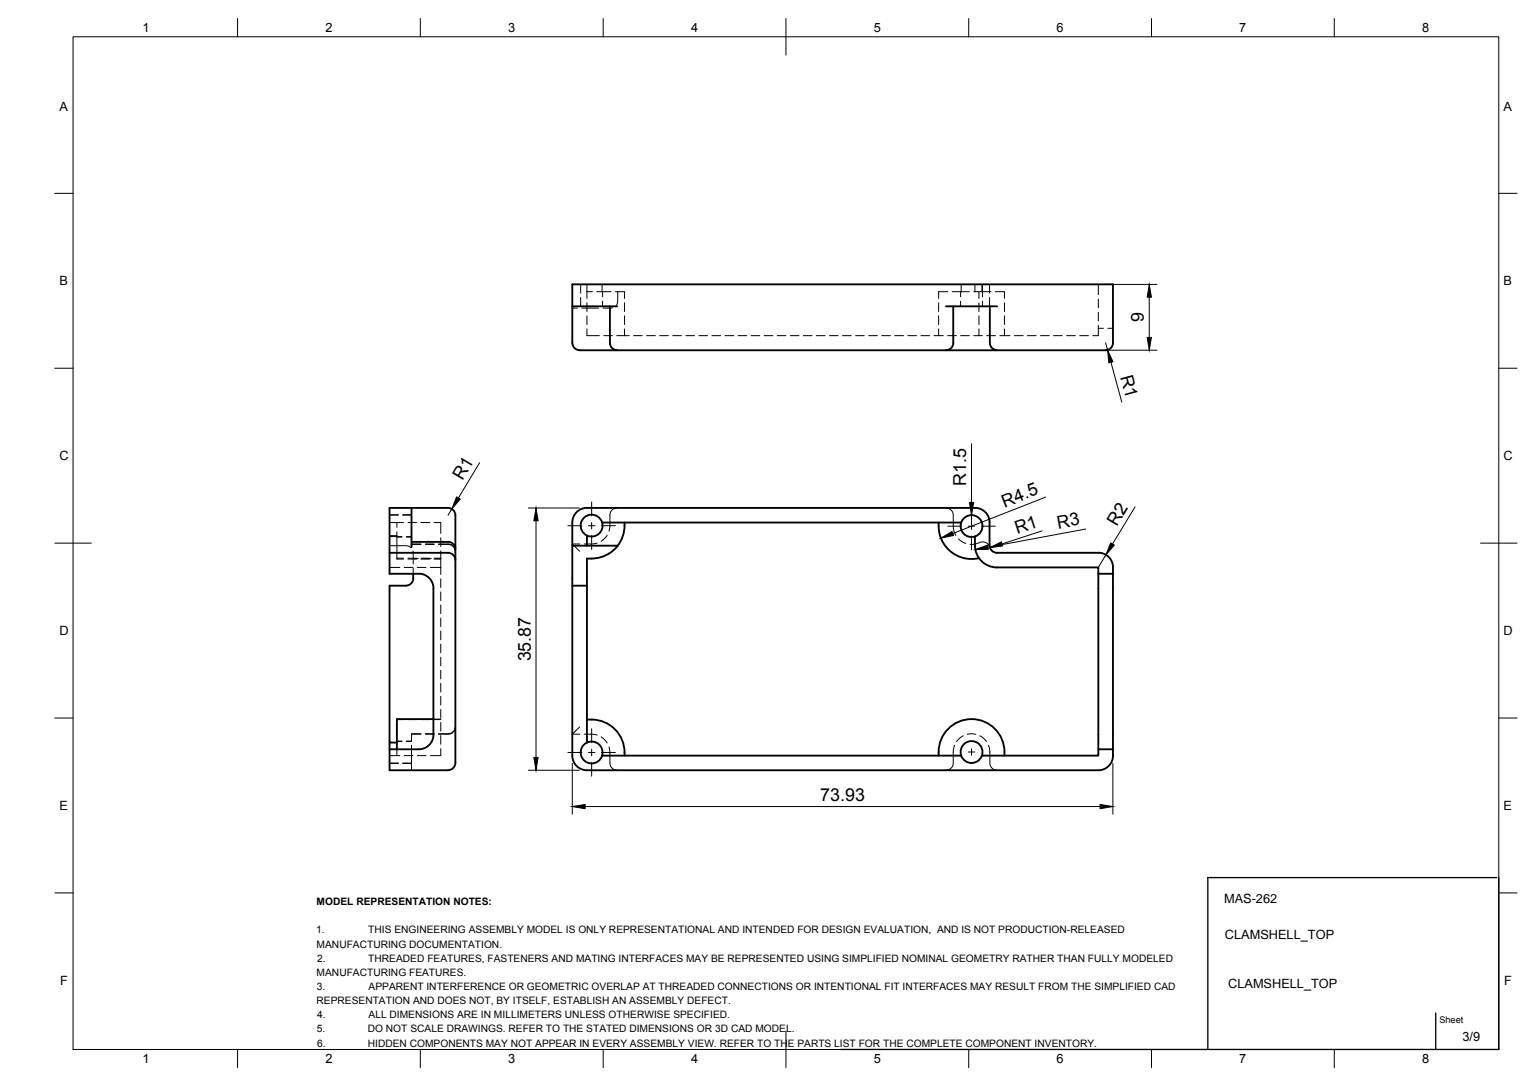
ISO-10303-21;
HEADER;
/* Generated by software containing ST-Developer
 * from STEP Tools, Inc. (www.steptools.com) 
 */

FILE_DESCRIPTION(
/* description */ (''),
/* implementation_level */ '2;1');

FILE_NAME(
/* name */ 'CLAMSHELL_TOP.step',
/* time_stamp */ '2026-10-07T02:13:48+06:00',
/* author */ (''),
/* organization */ (''),
/* preprocessor_version */ 'ST-DEVELOPER v20.2',
/* originating_system */ 'Autodesk Translation Framework v15.15.0.0',
/* authorisation */ '');

FILE_SCHEMA (('AUTOMOTIVE_DESIGN { 1 0 10303 214 3 1 1 }'));
ENDSEC;

DATA;
#10=MECHANICAL_DESIGN_GEOMETRIC_PRESENTATION_REPRESENTATION('',(#114),#17042);
#90=SHAPE_REPRESENTATION_RELATIONSHIP('SRR','None',#17086,#102);
#102=ADVANCED_BREP_SHAPE_REPRESENTATION('',(#126),#17030);
#114=STYLED_ITEM('',(#17154),#126);
#126=MANIFOLD_SOLID_BREP('Body1',#8115);
#138=FACE_BOUND('',#1043,.T.);
#139=FACE_BOUND('',#1045,.T.);
#140=FACE_BOUND('',#1050,.T.);
#141=FACE_BOUND('',#1052,.T.);
#178=(
BOUNDED_SURFACE()
B_SPLINE_SURFACE(2,2,((#12260,#12261,#12262),(#12263,#12264,#12265),(#12266,
#12267,#12268)),.UNSPECIFIED.,.F.,.F.,.F.)
B_SPLINE_SURFACE_WITH_KNOTS((3,3),(3,3),(-1.5707963267949,0.),(0.,1.5707963267949),
 .UNSPECIFIED.)
GEOMETRIC_REPRESENTATION_ITEM()
RATIONAL_B_SPLINE_SURFACE(((1.,0.707106781186548,1.),(0.707106781186558,
0.500000000000007,0.707106781186558),(1.,0.707106781186548,1.)))
REPRESENTATION_ITEM('')
SURFACE()
);
#179=(
BOUNDED_SURFACE()
B_SPLINE_SURFACE(2,2,((#12273,#12274,#12275),(#12276,#12277,#12278),(#12279,
#12280,#12281)),.UNSPECIFIED.,.F.,.F.,.F.)
B_SPLINE_SURFACE_WITH_KNOTS((3,3),(3,3),(-1.5707963267949,0.),(-1.5707963267949,
0.),.UNSPECIFIED.)
GEOMETRIC_REPRESENTATION_ITEM()
RATIONAL_B_SPLINE_SURFACE(((1.,0.707106781186548,1.),(0.707106781186552,
0.500000000000003,0.707106781186552),(1.,0.707106781186548,1.)))
REPRESENTATION_ITEM('')
SURFACE()
);
#196=SPHERICAL_SURFACE('',#8306,1.);
#197=SPHERICAL_SURFACE('',#8311,1.);
#198=SPHERICAL_SURFACE('',#8414,1.);
#199=SPHERICAL_SURFACE('',#8416,1.);
#200=SPHERICAL_SURFACE('',#8418,1.);
#201=SPHERICAL_SURFACE('',#8420,1.);
#214=TOROIDAL_SURFACE('',#8295,3.5,1.);
#215=TOROIDAL_SURFACE('',#8300,3.5,1.);
#216=TOROIDAL_SURFACE('',#8389,3.5,1.);
#217=TOROIDAL_SURFACE('',#8394,2.,1.);
#218=TOROIDAL_SURFACE('',#8411,3.5,1.);
#237=ELLIPSE('',#8289,1.4142135623731,1.);
#238=ELLIPSE('',#8291,1.41421356237309,1.);
#284=PLANE('',#8266);
#285=PLANE('',#8267);
#286=PLANE('',#8270);
#287=PLANE('',#8274);
#288=PLANE('',#8275);
#289=PLANE('',#8276);
#290=PLANE('',#8277);
#291=PLANE('',#8313);
#292=PLANE('',#8316);
#293=PLANE('',#8324);
#294=PLANE('',#8325);
#295=PLANE('',#8326);
#296=PLANE('',#8330);
#297=PLANE('',#8334);
#298=PLANE('',#8335);
#299=PLANE('',#8357);
#300=PLANE('',#8358);
#301=PLANE('',#8359);
#302=PLANE('',#8361);
#303=PLANE('',#8362);
#304=PLANE('',#8363);
#305=PLANE('',#8364);
#306=PLANE('',#8365);
#307=PLANE('',#8370);
#308=PLANE('',#8375);
#309=PLANE('',#8376);
#310=PLANE('',#8377);
#311=PLANE('',#8378);
#312=PLANE('',#8380);
#313=PLANE('',#8381);
#314=PLANE('',#8384);
#315=PLANE('',#8385);
#316=PLANE('',#8424);
#317=PLANE('',#8427);
#318=PLANE('',#8432);
#319=PLANE('',#8439);
#320=PLANE('',#8442);
#321=PLANE('',#8443);
#322=PLANE('',#8446);
#323=PLANE('',#8448);
#324=PLANE('',#8450);
#325=PLANE('',#8453);
#326=PLANE('',#8454);
#327=PLANE('',#8456);
#328=PLANE('',#8457);
#329=PLANE('',#8458);
#476=FACE_OUTER_BOUND('',#953,.T.);
#477=FACE_OUTER_BOUND('',#954,.T.);
#478=FACE_OUTER_BOUND('',#955,.T.);
#479=FACE_OUTER_BOUND('',#956,.T.);
#480=FACE_OUTER_BOUND('',#957,.T.);
#481=FACE_OUTER_BOUND('',#958,.T.);
#482=FACE_OUTER_BOUND('',#959,.T.);
#483=FACE_OUTER_BOUND('',#960,.T.);
#484=FACE_OUTER_BOUND('',#961,.T.);
#485=FACE_OUTER_BOUND('',#962,.T.);
#486=FACE_OUTER_BOUND('',#963,.T.);
#487=FACE_OUTER_BOUND('',#964,.T.);
#488=FACE_OUTER_BOUND('',#965,.T.);
#489=FACE_OUTER_BOUND('',#966,.T.);
#490=FACE_OUTER_BOUND('',#967,.T.);
#491=FACE_OUTER_BOUND('',#968,.T.);
#492=FACE_OUTER_BOUND('',#969,.T.);
#493=FACE_OUTER_BOUND('',#970,.T.);
#494=FACE_OUTER_BOUND('',#971,.T.);
#495=FACE_OUTER_BOUND('',#972,.T.);
#496=FACE_OUTER_BOUND('',#973,.T.);
#497=FACE_OUTER_BOUND('',#974,.T.);
#498=FACE_OUTER_BOUND('',#975,.T.);
#499=FACE_OUTER_BOUND('',#976,.T.);
#500=FACE_OUTER_BOUND('',#977,.T.);
#501=FACE_OUTER_BOUND('',#978,.T.);
#502=FACE_OUTER_BOUND('',#979,.T.);
#503=FACE_OUTER_BOUND('',#980,.T.);
#504=FACE_OUTER_BOUND('',#981,.T.);
#505=FACE_OUTER_BOUND('',#982,.T.);
#506=FACE_OUTER_BOUND('',#983,.T.);
#507=FACE_OUTER_BOUND('',#984,.T.);
#508=FACE_OUTER_BOUND('',#985,.T.);
#509=FACE_OUTER_BOUND('',#986,.T.);
#510=FACE_OUTER_BOUND('',#987,.T.);
#511=FACE_OUTER_BOUND('',#988,.T.);
#512=FACE_OUTER_BOUND('',#989,.T.);
#513=FACE_OUTER_BOUND('',#990,.T.);
#514=FACE_OUTER_BOUND('',#991,.T.);
#515=FACE_OUTER_BOUND('',#992,.T.);
#516=FACE_OUTER_BOUND('',#993,.T.);
#517=FACE_OUTER_BOUND('',#994,.T.);
#518=FACE_OUTER_BOUND('',#995,.T.);
#519=FACE_OUTER_BOUND('',#996,.T.);
#520=FACE_OUTER_BOUND('',#997,.T.);
#521=FACE_OUTER_BOUND('',#998,.T.);
#522=FACE_OUTER_BOUND('',#999,.T.);
#523=FACE_OUTER_BOUND('',#1000,.T.);
#524=FACE_OUTER_BOUND('',#1001,.T.);
#525=FACE_OUTER_BOUND('',#1002,.T.);
#526=FACE_OUTER_BOUND('',#1003,.T.);
#527=FACE_OUTER_BOUND('',#1004,.T.);
#528=FACE_OUTER_BOUND('',#1005,.T.);
#529=FACE_OUTER_BOUND('',#1006,.T.);
#530=FACE_OUTER_BOUND('',#1007,.T.);
#531=FACE_OUTER_BOUND('',#1008,.T.);
#532=FACE_OUTER_BOUND('',#1009,.T.);
#533=FACE_OUTER_BOUND('',#1010,.T.);
#534=FACE_OUTER_BOUND('',#1011,.T.);
#535=FACE_OUTER_BOUND('',#1012,.T.);
#536=FACE_OUTER_BOUND('',#1013,.T.);
#537=FACE_OUTER_BOUND('',#1014,.T.);
#538=FACE_OUTER_BOUND('',#1015,.T.);
#539=FACE_OUTER_BOUND('',#1016,.T.);
#540=FACE_OUTER_BOUND('',#1017,.T.);
#541=FACE_OUTER_BOUND('',#1018,.T.);
#542=FACE_OUTER_BOUND('',#1019,.T.);
#543=FACE_OUTER_BOUND('',#1020,.T.);
#544=FACE_OUTER_BOUND('',#1021,.T.);
#545=FACE_OUTER_BOUND('',#1022,.T.);
#546=FACE_OUTER_BOUND('',#1023,.T.);
#547=FACE_OUTER_BOUND('',#1024,.T.);
#548=FACE_OUTER_BOUND('',#1025,.T.);
#549=FACE_OUTER_BOUND('',#1026,.T.);
#550=FACE_OUTER_BOUND('',#1027,.T.);
#551=FACE_OUTER_BOUND('',#1028,.T.);
#552=FACE_OUTER_BOUND('',#1029,.T.);
#553=FACE_OUTER_BOUND('',#1030,.T.);
#554=FACE_OUTER_BOUND('',#1031,.T.);
#555=FACE_OUTER_BOUND('',#1032,.T.);
#556=FACE_OUTER_BOUND('',#1033,.T.);
#557=FACE_OUTER_BOUND('',#1034,.T.);
#558=FACE_OUTER_BOUND('',#1035,.T.);
#559=FACE_OUTER_BOUND('',#1036,.T.);
#560=FACE_OUTER_BOUND('',#1037,.T.);
#561=FACE_OUTER_BOUND('',#1038,.T.);
#562=FACE_OUTER_BOUND('',#1039,.T.);
#563=FACE_OUTER_BOUND('',#1040,.T.);
#564=FACE_OUTER_BOUND('',#1041,.T.);
#565=FACE_OUTER_BOUND('',#1042,.T.);
#566=FACE_OUTER_BOUND('',#1044,.T.);
#567=FACE_OUTER_BOUND('',#1046,.T.);
#568=FACE_OUTER_BOUND('',#1047,.T.);
#569=FACE_OUTER_BOUND('',#1048,.T.);
#570=FACE_OUTER_BOUND('',#1049,.T.);
#571=FACE_OUTER_BOUND('',#1051,.T.);
#572=FACE_OUTER_BOUND('',#1053,.T.);
#573=FACE_OUTER_BOUND('',#1054,.T.);
#574=FACE_OUTER_BOUND('',#1055,.T.);
#575=FACE_OUTER_BOUND('',#1056,.T.);
#576=FACE_OUTER_BOUND('',#1057,.T.);
#953=EDGE_LOOP('',(#5089,#5090,#5091,#5092,#5093,#5094,#5095));
#954=EDGE_LOOP('',(#5096,#5097,#5098,#5099));
#955=EDGE_LOOP('',(#5100,#5101,#5102,#5103,#5104,#5105));
#956=EDGE_LOOP('',(#5106,#5107,#5108,#5109));
#957=EDGE_LOOP('',(#5110,#5111,#5112,#5113,#5114,#5115));
#958=EDGE_LOOP('',(#5116,#5117,#5118,#5119));
#959=EDGE_LOOP('',(#5120,#5121,#5122,#5123));
#960=EDGE_LOOP('',(#5124,#5125,#5126,#5127));
#961=EDGE_LOOP('',(#5128,#5129,#5130,#5131,#5132,#5133,#5134,#5135,#5136));
#962=EDGE_LOOP('',(#5137,#5138,#5139,#5140,#5141,#5142,#5143,#5144,#5145,
#5146,#5147,#5148,#5149,#5150,#5151));
#963=EDGE_LOOP('',(#5152,#5153,#5154,#5155));
#964=EDGE_LOOP('',(#5156,#5157,#5158,#5159));
#965=EDGE_LOOP('',(#5160,#5161,#5162,#5163));
#966=EDGE_LOOP('',(#5164,#5165,#5166,#5167));
#967=EDGE_LOOP('',(#5168,#5169,#5170,#5171));
#968=EDGE_LOOP('',(#5172,#5173,#5174,#5175));
#969=EDGE_LOOP('',(#5176,#5177,#5178,#5179));
#970=EDGE_LOOP('',(#5180,#5181,#5182,#5183));
#971=EDGE_LOOP('',(#5184,#5185,#5186));
#972=EDGE_LOOP('',(#5187,#5188,#5189,#5190));
#973=EDGE_LOOP('',(#5191,#5192,#5193));
#974=EDGE_LOOP('',(#5194,#5195,#5196,#5197,#5198,#5199,#5200,#5201,#5202,
#5203));
#975=EDGE_LOOP('',(#5204,#5205,#5206,#5207));
#976=EDGE_LOOP('',(#5208,#5209,#5210,#5211,#5212,#5213,#5214,#5215,#5216,
#5217,#5218,#5219,#5220,#5221,#5222,#5223,#5224,#5225,#5226,#5227));
#977=EDGE_LOOP('',(#5228,#5229,#5230,#5231));
#978=EDGE_LOOP('',(#5232,#5233,#5234,#5235,#5236,#5237,#5238,#5239));
#979=EDGE_LOOP('',(#5240,#5241,#5242,#5243));
#980=EDGE_LOOP('',(#5244,#5245,#5246,#5247));
#981=EDGE_LOOP('',(#5248,#5249,#5250,#5251));
#982=EDGE_LOOP('',(#5252,#5253,#5254,#5255));
#983=EDGE_LOOP('',(#5256,#5257,#5258,#5259));
#984=EDGE_LOOP('',(#5260,#5261,#5262,#5263,#5264,#5265,#5266,#5267,#5268,
#5269));
#985=EDGE_LOOP('',(#5270,#5271,#5272,#5273,#5274,#5275,#5276,#5277,#5278,
#5279,#5280,#5281,#5282,#5283,#5284,#5285,#5286,#5287,#5288));
#986=EDGE_LOOP('',(#5289,#5290,#5291,#5292,#5293,#5294,#5295,#5296));
#987=EDGE_LOOP('',(#5297,#5298,#5299,#5300,#5301,#5302,#5303,#5304));
#988=EDGE_LOOP('',(#5305,#5306,#5307,#5308,#5309,#5310,#5311,#5312));
#989=EDGE_LOOP('',(#5313,#5314,#5315,#5316,#5317,#5318,#5319,#5320));
#990=EDGE_LOOP('',(#5321,#5322,#5323,#5324));
#991=EDGE_LOOP('',(#5325,#5326,#5327,#5328,#5329,#5330,#5331));
#992=EDGE_LOOP('',(#5332,#5333,#5334,#5335,#5336,#5337));
#993=EDGE_LOOP('',(#5338,#5339,#5340,#5341,#5342,#5343));
#994=EDGE_LOOP('',(#5344,#5345,#5346,#5347,#5348,#5349,#5350,#5351));
#995=EDGE_LOOP('',(#5352,#5353,#5354,#5355));
#996=EDGE_LOOP('',(#5356,#5357,#5358,#5359,#5360,#5361,#5362,#5363,#5364,
#5365));
#997=EDGE_LOOP('',(#5366,#5367,#5368,#5369,#5370,#5371,#5372,#5373,#5374,
#5375,#5376,#5377,#5378,#5379,#5380,#5381,#5382,#5383));
#998=EDGE_LOOP('',(#5384,#5385,#5386,#5387));
#999=EDGE_LOOP('',(#5388,#5389,#5390,#5391,#5392,#5393));
#1000=EDGE_LOOP('',(#5394,#5395,#5396,#5397));
#1001=EDGE_LOOP('',(#5398,#5399,#5400,#5401));
#1002=EDGE_LOOP('',(#5402,#5403,#5404,#5405));
#1003=EDGE_LOOP('',(#5406,#5407,#5408,#5409,#5410,#5411,#5412));
#1004=EDGE_LOOP('',(#5413,#5414,#5415,#5416,#5417,#5418,#5419,#5420));
#1005=EDGE_LOOP('',(#5421,#5422,#5423,#5424));
#1006=EDGE_LOOP('',(#5425,#5426,#5427,#5428));
#1007=EDGE_LOOP('',(#5429,#5430,#5431,#5432));
#1008=EDGE_LOOP('',(#5433,#5434,#5435,#5436));
#1009=EDGE_LOOP('',(#5437,#5438,#5439,#5440,#5441,#5442));
#1010=EDGE_LOOP('',(#5443,#5444,#5445,#5446));
#1011=EDGE_LOOP('',(#5447,#5448,#5449,#5450));
#1012=EDGE_LOOP('',(#5451,#5452,#5453,#5454));
#1013=EDGE_LOOP('',(#5455,#5456,#5457,#5458));
#1014=EDGE_LOOP('',(#5459,#5460,#5461,#5462));
#1015=EDGE_LOOP('',(#5463,#5464,#5465,#5466));
#1016=EDGE_LOOP('',(#5467,#5468,#5469,#5470));
#1017=EDGE_LOOP('',(#5471,#5472,#5473,#5474));
#1018=EDGE_LOOP('',(#5475,#5476,#5477,#5478));
#1019=EDGE_LOOP('',(#5479,#5480,#5481,#5482));
#1020=EDGE_LOOP('',(#5483,#5484,#5485,#5486));
#1021=EDGE_LOOP('',(#5487,#5488,#5489,#5490));
#1022=EDGE_LOOP('',(#5491,#5492,#5493));
#1023=EDGE_LOOP('',(#5494,#5495,#5496));
#1024=EDGE_LOOP('',(#5497,#5498,#5499));
#1025=EDGE_LOOP('',(#5500,#5501,#5502));
#1026=EDGE_LOOP('',(#5503,#5504,#5505,#5506));
#1027=EDGE_LOOP('',(#5507,#5508,#5509,#5510));
#1028=EDGE_LOOP('',(#5511,#5512,#5513,#5514));
#1029=EDGE_LOOP('',(#5515,#5516,#5517,#5518));
#1030=EDGE_LOOP('',(#5519,#5520,#5521,#5522));
#1031=EDGE_LOOP('',(#5523,#5524,#5525,#5526));
#1032=EDGE_LOOP('',(#5527,#5528,#5529,#5530));
#1033=EDGE_LOOP('',(#5531,#5532,#5533,#5534));
#1034=EDGE_LOOP('',(#5535,#5536,#5537,#5538,#5539,#5540));
#1035=EDGE_LOOP('',(#5541,#5542,#5543,#5544));
#1036=EDGE_LOOP('',(#5545,#5546,#5547,#5548));
#1037=EDGE_LOOP('',(#5549,#5550,#5551,#5552));
#1038=EDGE_LOOP('',(#5553,#5554,#5555,#5556));
#1039=EDGE_LOOP('',(#5557,#5558,#5559,#5560));
#1040=EDGE_LOOP('',(#5561,#5562,#5563,#5564));
#1041=EDGE_LOOP('',(#5565,#5566,#5567,#5568));
#1042=EDGE_LOOP('',(#5569,#5570,#5571,#5572,#5573,#5574,#5575));
#1043=EDGE_LOOP('',(#5576));
#1044=EDGE_LOOP('',(#5577,#5578,#5579,#5580,#5581,#5582,#5583,#5584));
#1045=EDGE_LOOP('',(#5585));
#1046=EDGE_LOOP('',(#5586,#5587,#5588,#5589));
#1047=EDGE_LOOP('',(#5590,#5591,#5592,#5593));
#1048=EDGE_LOOP('',(#5594,#5595,#5596,#5597));
#1049=EDGE_LOOP('',(#5598,#5599,#5600,#5601,#5602,#5603,#5604));
#1050=EDGE_LOOP('',(#5605));
#1051=EDGE_LOOP('',(#5606,#5607,#5608,#5609,#5610,#5611));
#1052=EDGE_LOOP('',(#5612));
#1053=EDGE_LOOP('',(#5613,#5614,#5615,#5616));
#1054=EDGE_LOOP('',(#5617,#5618,#5619,#5620,#5621,#5622,#5623,#5624,#5625,
#5626,#5627,#5628,#5629,#5630));
#1055=EDGE_LOOP('',(#5631,#5632,#5633,#5634));
#1056=EDGE_LOOP('',(#5635,#5636,#5637,#5638));
#1057=EDGE_LOOP('',(#5639,#5640,#5641,#5642));
#1470=CIRCLE('',#8263,4.5);
#1471=CIRCLE('',#8264,4.5);
#1472=CIRCLE('',#8265,4.5);
#1473=CIRCLE('',#8269,1.);
#1474=CIRCLE('',#8272,0.999999999999998);
#1475=CIRCLE('',#8273,0.999999999999998);
#1476=CIRCLE('',#8278,2.);
#1477=CIRCLE('',#8279,2.);
#1478=CIRCLE('',#8280,1.5);
#1479=CIRCLE('',#8281,1.5);
#1480=CIRCLE('',#8282,1.5);
#1481=CIRCLE('',#8283,1.5);
#1482=CIRCLE('',#8285,0.999999999999999);
#1483=CIRCLE('',#8286,1.);
#1484=CIRCLE('',#8288,1.);
#1485=CIRCLE('',#8293,1.);
#1486=CIRCLE('',#8294,0.999999999999999);
#1487=CIRCLE('',#8296,1.);
#1488=CIRCLE('',#8297,3.5);
#1489=CIRCLE('',#8298,2.5);
#1490=CIRCLE('',#8301,1.);
#1491=CIRCLE('',#8302,3.5);
#1492=CIRCLE('',#8303,2.5);
#1493=CIRCLE('',#8305,0.999999999999999);
#1494=CIRCLE('',#8307,1.);
#1495=CIRCLE('',#8309,1.);
#1496=CIRCLE('',#8310,1.);
#1497=CIRCLE('',#8312,1.);
#1498=CIRCLE('',#8315,1.);
#1499=CIRCLE('',#8317,3.5);
#1500=CIRCLE('',#8318,2.);
#1501=CIRCLE('',#8319,1.);
#1502=CIRCLE('',#8320,1.);
#1503=CIRCLE('',#8321,3.5);
#1504=CIRCLE('',#8323,1.);
#1505=CIRCLE('',#8328,2.);
#1506=CIRCLE('',#8329,2.);
#1507=CIRCLE('',#8332,2.);
#1508=CIRCLE('',#8333,2.);
#1509=CIRCLE('',#8336,1.5);
#1510=CIRCLE('',#8337,1.5);
#1511=CIRCLE('',#8338,3.);
#1512=CIRCLE('',#8339,2.);
#1513=CIRCLE('',#8340,0.999999999999996);
#1514=CIRCLE('',#8341,2.);
#1515=CIRCLE('',#8342,2.);
#1516=CIRCLE('',#8344,1.5);
#1517=CIRCLE('',#8345,1.5);
#1518=CIRCLE('',#8346,1.5);
#1519=CIRCLE('',#8348,1.5);
#1520=CIRCLE('',#8349,1.5);
#1521=CIRCLE('',#8350,1.5);
#1522=CIRCLE('',#8352,1.5);
#1523=CIRCLE('',#8353,1.5);
#1524=CIRCLE('',#8355,1.5);
#1525=CIRCLE('',#8356,1.5);
#1526=CIRCLE('',#8360,4.5);
#1527=CIRCLE('',#8366,4.5);
#1528=CIRCLE('',#8367,4.5);
#1529=CIRCLE('',#8368,4.5);
#1530=CIRCLE('',#8369,3.);
#1531=CIRCLE('',#8372,3.);
#1532=CIRCLE('',#8374,4.5);
#1533=CIRCLE('',#8383,4.5);
#1534=CIRCLE('',#8387,1.);
#1535=CIRCLE('',#8388,0.999999999999996);
#1536=CIRCLE('',#8390,0.999999999999996);
#1537=CIRCLE('',#8391,2.5);
#1538=CIRCLE('',#8393,0.999999999999996);
#1539=CIRCLE('',#8395,1.);
#1540=CIRCLE('',#8396,0.999999999999996);
#1541=CIRCLE('',#8397,1.);
#1542=CIRCLE('',#8399,1.);
#1543=CIRCLE('',#8400,1.00000000000001);
#1544=CIRCLE('',#8401,2.);
#1545=CIRCLE('',#8403,0.999999999999996);
#1546=CIRCLE('',#8404,1.);
#1547=CIRCLE('',#8405,2.);
#1548=CIRCLE('',#8407,1.);
#1549=CIRCLE('',#8409,1.);
#1550=CIRCLE('',#8410,0.999999999999996);
#1551=CIRCLE('',#8412,1.);
#1552=CIRCLE('',#8413,2.5);
#1553=CIRCLE('',#8415,0.999999999999998);
#1554=CIRCLE('',#8417,1.);
#1555=CIRCLE('',#8419,1.);
#1556=CIRCLE('',#8421,1.);
#1557=CIRCLE('',#8423,1.);
#1558=CIRCLE('',#8426,2.5);
#1559=CIRCLE('',#8429,1.);
#1560=CIRCLE('',#8434,0.999999999999996);
#1561=CIRCLE('',#8436,1.);
#1562=CIRCLE('',#8438,2.5);
#1563=CIRCLE('',#8441,1.);
#1564=CIRCLE('',#8445,2.5);
#1565=CIRCLE('',#8447,2.);
#1566=CIRCLE('',#8449,2.);
#1567=CIRCLE('',#8452,2.5);
#1568=CIRCLE('',#8455,2.);
#1950=B_SPLINE_CURVE_WITH_KNOTS('',3,(#11818,#11819,#11820,#11821,#11822,
#11823,#11824,#11825,#11826,#11827,#11828,#11829),.UNSPECIFIED.,.F.,.F.,
(4,2,2,2,2,4),(0.684266710157815,0.698356622095572,0.712446534033328,0.731803474638004,
0.751160415242679,0.78032220184246),.UNSPECIFIED.);
#2022=LINE('',#11816,#2600);
#2023=LINE('',#11833,#2601);
#2024=LINE('',#11837,#2602);
#2025=LINE('',#11841,#2603);
#2026=LINE('',#11843,#2604);
#2027=LINE('',#11844,#2605);
#2028=LINE('',#11848,#2606);
#2029=LINE('',#11850,#2607);
#2030=LINE('',#11851,#2608);
#2031=LINE('',#11853,#2609);
#2032=LINE('',#11854,#2610);
#2033=LINE('',#11858,#2611);
#2034=LINE('',#11861,#2612);
#2035=LINE('',#11863,#2613);
#2036=LINE('',#11864,#2614);
#2037=LINE('',#11869,#2615);
#2038=LINE('',#11874,#2616);
#2039=LINE('',#11875,#2617);
#2040=LINE('',#11876,#2618);
#2041=LINE('',#11879,#2619);
#2042=LINE('',#11881,#2620);
#2043=LINE('',#11882,#2621);
#2044=LINE('',#11885,#2622);
#2045=LINE('',#11887,#2623);
#2046=LINE('',#11889,#2624);
#2047=LINE('',#11891,#2625);
#2048=LINE('',#11892,#2626);
#2049=LINE('',#11895,#2627);
#2050=LINE('',#11899,#2628);
#2051=LINE('',#11903,#2629);
#2052=LINE('',#11905,#2630);
#2053=LINE('',#11907,#2631);
#2054=LINE('',#11909,#2632);
#2055=LINE('',#11915,#2633);
#2056=LINE('',#11924,#2634);
#2057=LINE('',#11927,#2635);
#2058=LINE('',#11931,#2636);
#2059=LINE('',#11935,#2637);
#2060=LINE('',#11939,#2638);
#2061=LINE('',#11942,#2639);
#2062=LINE('',#11947,#2640);
#2063=LINE('',#11950,#2641);
#2064=LINE('',#11958,#2642);
#2065=LINE('',#11959,#2643);
#2066=LINE('',#11970,#2644);
#2067=LINE('',#11971,#2645);
#2068=LINE('',#11978,#2646);
#2069=LINE('',#11981,#2647);
#2070=LINE('',#11986,#2648);
#2071=LINE('',#11988,#2649);
#2072=LINE('',#11990,#2650);
#2073=LINE('',#11992,#2651);
#2074=LINE('',#11994,#2652);
#2075=LINE('',#11996,#2653);
#2076=LINE('',#11997,#2654);
#2077=LINE('',#11998,#2655);
#2078=LINE('',#12001,#2656);
#2079=LINE('',#12005,#2657);
#2080=LINE('',#12007,#2658);
#2081=LINE('',#12013,#2659);
#2082=LINE('',#12017,#2660);
#2083=LINE('',#12021,#2661);
#2084=LINE('',#12023,#2662);
#2085=LINE('',#12026,#2663);
#2086=LINE('',#12029,#2664);
#2087=LINE('',#12033,#2665);
#2088=LINE('',#12035,#2666);
#2089=LINE('',#12037,#2667);
#2090=LINE('',#12039,#2668);
#2091=LINE('',#12041,#2669);
#2092=LINE('',#12042,#2670);
#2093=LINE('',#12046,#2671);
#2094=LINE('',#12048,#2672);
#2095=LINE('',#12050,#2673);
#2096=LINE('',#12051,#2674);
#2097=LINE('',#12055,#2675);
#2098=LINE('',#12057,#2676);
#2099=LINE('',#12059,#2677);
#2100=LINE('',#12060,#2678);
#2101=LINE('',#12066,#2679);
#2102=LINE('',#12068,#2680);
#2103=LINE('',#12069,#2681);
#2104=LINE('',#12075,#2682);
#2105=LINE('',#12077,#2683);
#2106=LINE('',#12079,#2684);
#2107=LINE('',#12080,#2685);
#2108=LINE('',#12085,#2686);
#2109=LINE('',#12089,#2687);
#2110=LINE('',#12093,#2688);
#2111=LINE('',#12094,#2689);
#2112=LINE('',#12098,#2690);
#2113=LINE('',#12102,#2691);
#2114=LINE('',#12106,#2692);
#2115=LINE('',#12111,#2693);
#2116=LINE('',#12114,#2694);
#2117=LINE('',#12116,#2695);
#2118=LINE('',#12122,#2696);
#2119=LINE('',#12125,#2697);
#2120=LINE('',#12130,#2698);
#2121=LINE('',#12132,#2699);
#2122=LINE('',#12135,#2700);
#2123=LINE('',#12139,#2701);
#2124=LINE('',#12141,#2702);
#2125=LINE('',#12145,#2703);
#2126=LINE('',#12146,#2704);
#2127=LINE('',#12149,#2705);
#2128=LINE('',#12150,#2706);
#2129=LINE('',#12153,#2707);
#2130=LINE('',#12155,#2708);
#2131=LINE('',#12159,#2709);
#2132=LINE('',#12160,#2710);
#2133=LINE('',#12163,#2711);
#2134=LINE('',#12165,#2712);
#2135=LINE('',#12166,#2713);
#2136=LINE('',#12169,#2714);
#2137=LINE('',#12171,#2715);
#2138=LINE('',#12173,#2716);
#2139=LINE('',#12174,#2717);
#2140=LINE('',#12177,#2718);
#2141=LINE('',#12178,#2719);
#2142=LINE('',#12181,#2720);
#2143=LINE('',#12182,#2721);
#2144=LINE('',#12188,#2722);
#2145=LINE('',#12190,#2723);
#2146=LINE('',#12191,#2724);
#2147=LINE('',#12193,#2725);
#2148=LINE('',#12196,#2726);
#2149=LINE('',#12198,#2727);
#2150=LINE('',#12201,#2728);
#2151=LINE('',#12204,#2729);
#2152=LINE('',#12208,#2730);
#2153=LINE('',#12212,#2731);
#2154=LINE('',#12214,#2732);
#2155=LINE('',#12217,#2733);
#2156=LINE('',#12218,#2734);
#2157=LINE('',#12220,#2735);
#2158=LINE('',#12222,#2736);
#2159=LINE('',#12226,#2737);
#2160=LINE('',#12227,#2738);
#2161=LINE('',#12230,#2739);
#2162=LINE('',#12231,#2740);
#2163=LINE('',#12240,#2741);
#2164=LINE('',#12249,#2742);
#2165=LINE('',#12259,#2743);
#2166=LINE('',#12290,#2744);
#2167=LINE('',#12306,#2745);
#2168=LINE('',#12310,#2746);
#2169=LINE('',#12311,#2747);
#2170=LINE('',#12314,#2748);
#2171=LINE('',#12318,#2749);
#2172=LINE('',#12319,#2750);
#2173=LINE('',#12324,#2751);
#2174=LINE('',#12326,#2752);
#2175=LINE('',#12329,#2753);
#2176=LINE('',#12332,#2754);
#2177=LINE('',#12335,#2755);
#2178=LINE('',#12339,#2756);
#2179=LINE('',#12343,#2757);
#2180=LINE('',#12344,#2758);
#2181=LINE('',#12349,#2759);
#2182=LINE('',#12350,#2760);
#2183=LINE('',#12353,#2761);
#2184=LINE('',#12355,#2762);
#2185=LINE('',#12356,#2763);
#2186=LINE('',#12362,#2764);
#2187=LINE('',#12365,#2765);
#2188=LINE('',#12369,#2766);
#2189=LINE('',#12370,#2767);
#2190=LINE('',#12373,#2768);
#2191=LINE('',#12377,#2769);
#2192=LINE('',#12378,#2770);
#2193=LINE('',#12381,#2771);
#2194=LINE('',#12385,#2772);
#2195=LINE('',#12387,#2773);
#2196=LINE('',#12388,#2774);
#2600=VECTOR('',#9257,20.);
#2601=VECTOR('',#9260,20.);
#2602=VECTOR('',#9263,20.);
#2603=VECTOR('',#9268,20.);
#2604=VECTOR('',#9269,20.);
#2605=VECTOR('',#9270,20.);
#2606=VECTOR('',#9273,20.);
#2607=VECTOR('',#9274,20.);
#2608=VECTOR('',#9275,20.);
#2609=VECTOR('',#9276,20.);
#2610=VECTOR('',#9277,20.);
#2611=VECTOR('',#9282,20.);
#2612=VECTOR('',#9285,20.);
#2613=VECTOR('',#9286,20.);
#2614=VECTOR('',#9287,20.);
#2615=VECTOR('',#9292,20.);
#2616=VECTOR('',#9297,20.);
#2617=VECTOR('',#9298,20.);
#2618=VECTOR('',#9299,20.);
#2619=VECTOR('',#9302,20.);
#2620=VECTOR('',#9303,20.);
#2621=VECTOR('',#9304,20.);
#2622=VECTOR('',#9307,20.);
#2623=VECTOR('',#9308,20.);
#2624=VECTOR('',#9309,20.);
#2625=VECTOR('',#9310,20.);
#2626=VECTOR('',#9311,20.);
#2627=VECTOR('',#9314,20.);
#2628=VECTOR('',#9317,20.);
#2629=VECTOR('',#9320,20.);
#2630=VECTOR('',#9321,20.);
#2631=VECTOR('',#9322,20.);
#2632=VECTOR('',#9323,20.);
#2633=VECTOR('',#9328,20.);
#2634=VECTOR('',#9337,20.);
#2635=VECTOR('',#9340,20.);
#2636=VECTOR('',#9343,20.);
#2637=VECTOR('',#9346,20.);
#2638=VECTOR('',#9351,20.);
#2639=VECTOR('',#9354,20.);
#2640=VECTOR('',#9359,20.);
#2641=VECTOR('',#9362,20.);
#2642=VECTOR('',#9373,20.);
#2643=VECTOR('',#9374,20.);
#2644=VECTOR('',#9387,20.);
#2645=VECTOR('',#9388,20.);
#2646=VECTOR('',#9397,20.);
#2647=VECTOR('',#9400,20.);
#2648=VECTOR('',#9407,20.);
#2649=VECTOR('',#9408,20.);
#2650=VECTOR('',#9409,20.);
#2651=VECTOR('',#9410,20.);
#2652=VECTOR('',#9411,20.);
#2653=VECTOR('',#9412,20.);
#2654=VECTOR('',#9413,20.);
#2655=VECTOR('',#9414,20.);
#2656=VECTOR('',#9417,20.);
#2657=VECTOR('',#9422,20.);
#2658=VECTOR('',#9423,20.);
#2659=VECTOR('',#9428,20.);
#2660=VECTOR('',#9431,20.);
#2661=VECTOR('',#9434,20.);
#2662=VECTOR('',#9435,20.);
#2663=VECTOR('',#9438,20.);
#2664=VECTOR('',#9441,20.);
#2665=VECTOR('',#9446,20.);
#2666=VECTOR('',#9447,20.);
#2667=VECTOR('',#9448,20.);
#2668=VECTOR('',#9449,20.);
#2669=VECTOR('',#9450,20.);
#2670=VECTOR('',#9451,20.);
#2671=VECTOR('',#9454,20.);
#2672=VECTOR('',#9455,20.);
#2673=VECTOR('',#9456,20.);
#2674=VECTOR('',#9457,20.);
#2675=VECTOR('',#9460,20.);
#2676=VECTOR('',#9461,20.);
#2677=VECTOR('',#9462,20.);
#2678=VECTOR('',#9463,20.);
#2679=VECTOR('',#9472,20.);
#2680=VECTOR('',#9473,20.);
#2681=VECTOR('',#9474,20.);
#2682=VECTOR('',#9483,20.);
#2683=VECTOR('',#9484,20.);
#2684=VECTOR('',#9485,20.);
#2685=VECTOR('',#9486,20.);
#2686=VECTOR('',#9491,20.);
#2687=VECTOR('',#9494,20.);
#2688=VECTOR('',#9497,20.);
#2689=VECTOR('',#9498,20.);
#2690=VECTOR('',#9501,20.);
#2691=VECTOR('',#9504,20.);
#2692=VECTOR('',#9509,20.);
#2693=VECTOR('',#9514,1.5);
#2694=VECTOR('',#9517,20.);
#2695=VECTOR('',#9518,20.);
#2696=VECTOR('',#9525,1.5);
#2697=VECTOR('',#9528,20.);
#2698=VECTOR('',#9535,1.5);
#2699=VECTOR('',#9536,20.);
#2700=VECTOR('',#9539,20.);
#2701=VECTOR('',#9544,1.5);
#2702=VECTOR('',#9545,20.);
#2703=VECTOR('',#9550,20.);
#2704=VECTOR('',#9551,20.);
#2705=VECTOR('',#9554,20.);
#2706=VECTOR('',#9555,20.);
#2707=VECTOR('',#9558,20.);
#2708=VECTOR('',#9559,20.);
#2709=VECTOR('',#9562,20.);
#2710=VECTOR('',#9563,20.);
#2711=VECTOR('',#9566,20.);
#2712=VECTOR('',#9567,20.);
#2713=VECTOR('',#9568,20.);
#2714=VECTOR('',#9571,20.);
#2715=VECTOR('',#9572,20.);
#2716=VECTOR('',#9573,20.);
#2717=VECTOR('',#9574,20.);
#2718=VECTOR('',#9577,20.);
#2719=VECTOR('',#9578,20.);
#2720=VECTOR('',#9581,20.);
#2721=VECTOR('',#9582,20.);
#2722=VECTOR('',#9587,20.);
#2723=VECTOR('',#9588,20.);
#2724=VECTOR('',#9589,20.);
#2725=VECTOR('',#9590,20.);
#2726=VECTOR('',#9593,20.);
#2727=VECTOR('',#9594,20.);
#2728=VECTOR('',#9597,20.);
#2729=VECTOR('',#9602,20.);
#2730=VECTOR('',#9607,20.);
#2731=VECTOR('',#9612,20.);
#2732=VECTOR('',#9615,20.);
#2733=VECTOR('',#9618,20.);
#2734=VECTOR('',#9619,20.);
#2735=VECTOR('',#9622,20.);
#2736=VECTOR('',#9625,20.);
#2737=VECTOR('',#9630,20.);
#2738=VECTOR('',#9631,20.);
#2739=VECTOR('',#9634,20.);
#2740=VECTOR('',#9635,20.);
#2741=VECTOR('',#9648,20.);
#2742=VECTOR('',#9661,20.);
#2743=VECTOR('',#9674,20.);
#2744=VECTOR('',#9695,20.);
#2745=VECTOR('',#9722,20.);
#2746=VECTOR('',#9727,20.);
#2747=VECTOR('',#9728,20.);
#2748=VECTOR('',#9731,20.);
#2749=VECTOR('',#9736,20.);
#2750=VECTOR('',#9737,20.);
#2751=VECTOR('',#9746,20.);
#2752=VECTOR('',#9749,20.);
#2753=VECTOR('',#9752,1.);
#2754=VECTOR('',#9755,20.);
#2755=VECTOR('',#9758,1.);
#2756=VECTOR('',#9763,20.);
#2757=VECTOR('',#9768,20.);
#2758=VECTOR('',#9769,20.);
#2759=VECTOR('',#9776,20.);
#2760=VECTOR('',#9777,20.);
#2761=VECTOR('',#9780,20.);
#2762=VECTOR('',#9781,20.);
#2763=VECTOR('',#9782,20.);
#2764=VECTOR('',#9791,20.);
#2765=VECTOR('',#9794,20.);
#2766=VECTOR('',#9799,20.);
#2767=VECTOR('',#9800,20.);
#2768=VECTOR('',#9803,20.);
#2769=VECTOR('',#9808,20.);
#2770=VECTOR('',#9809,20.);
#2771=VECTOR('',#9812,20.);
#2772=VECTOR('',#9819,20.);
#2773=VECTOR('',#9822,20.);
#2774=VECTOR('',#9823,20.);
#3178=VERTEX_POINT('',#11814);
#3179=VERTEX_POINT('',#11815);
#3180=VERTEX_POINT('',#11817);
#3181=VERTEX_POINT('',#11830);
#3182=VERTEX_POINT('',#11832);
#3183=VERTEX_POINT('',#11834);
#3184=VERTEX_POINT('',#11836);
#3185=VERTEX_POINT('',#11840);
#3186=VERTEX_POINT('',#11842);
#3187=VERTEX_POINT('',#11846);
#3188=VERTEX_POINT('',#11847);
#3189=VERTEX_POINT('',#11849);
#3190=VERTEX_POINT('',#11852);
#3191=VERTEX_POINT('',#11856);
#3192=VERTEX_POINT('',#11860);
#3193=VERTEX_POINT('',#11862);
#3194=VERTEX_POINT('',#11866);
#3195=VERTEX_POINT('',#11868);
#3196=VERTEX_POINT('',#11872);
#3197=VERTEX_POINT('',#11873);
#3198=VERTEX_POINT('',#11878);
#3199=VERTEX_POINT('',#11880);
#3200=VERTEX_POINT('',#11884);
#3201=VERTEX_POINT('',#11886);
#3202=VERTEX_POINT('',#11888);
#3203=VERTEX_POINT('',#11890);
#3204=VERTEX_POINT('',#11894);
#3205=VERTEX_POINT('',#11896);
#3206=VERTEX_POINT('',#11898);
#3207=VERTEX_POINT('',#11900);
#3208=VERTEX_POINT('',#11902);
#3209=VERTEX_POINT('',#11904);
#3210=VERTEX_POINT('',#11906);
#3211=VERTEX_POINT('',#11908);
#3212=VERTEX_POINT('',#11910);
#3213=VERTEX_POINT('',#11912);
#3214=VERTEX_POINT('',#11914);
#3215=VERTEX_POINT('',#11916);
#3216=VERTEX_POINT('',#11920);
#3217=VERTEX_POINT('',#11921);
#3218=VERTEX_POINT('',#11923);
#3219=VERTEX_POINT('',#11925);
#3220=VERTEX_POINT('',#11929);
#3221=VERTEX_POINT('',#11930);
#3222=VERTEX_POINT('',#11932);
#3223=VERTEX_POINT('',#11934);
#3224=VERTEX_POINT('',#11938);
#3225=VERTEX_POINT('',#11940);
#3226=VERTEX_POINT('',#11944);
#3227=VERTEX_POINT('',#11946);
#3228=VERTEX_POINT('',#11948);
#3229=VERTEX_POINT('',#11952);
#3230=VERTEX_POINT('',#11953);
#3231=VERTEX_POINT('',#11961);
#3232=VERTEX_POINT('',#11962);
#3233=VERTEX_POINT('',#11967);
#3234=VERTEX_POINT('',#11968);
#3235=VERTEX_POINT('',#11975);
#3236=VERTEX_POINT('',#11977);
#3237=VERTEX_POINT('',#11979);
#3238=VERTEX_POINT('',#11985);
#3239=VERTEX_POINT('',#11987);
#3240=VERTEX_POINT('',#11989);
#3241=VERTEX_POINT('',#11991);
#3242=VERTEX_POINT('',#11993);
#3243=VERTEX_POINT('',#11995);
#3244=VERTEX_POINT('',#12000);
#3245=VERTEX_POINT('',#12004);
#3246=VERTEX_POINT('',#12006);
#3247=VERTEX_POINT('',#12008);
#3248=VERTEX_POINT('',#12010);
#3249=VERTEX_POINT('',#12012);
#3250=VERTEX_POINT('',#12014);
#3251=VERTEX_POINT('',#12016);
#3252=VERTEX_POINT('',#12018);
#3253=VERTEX_POINT('',#12020);
#3254=VERTEX_POINT('',#12022);
#3255=VERTEX_POINT('',#12024);
#3256=VERTEX_POINT('',#12028);
#3257=VERTEX_POINT('',#12032);
#3258=VERTEX_POINT('',#12034);
#3259=VERTEX_POINT('',#12036);
#3260=VERTEX_POINT('',#12038);
#3261=VERTEX_POINT('',#12040);
#3262=VERTEX_POINT('',#12044);
#3263=VERTEX_POINT('',#12045);
#3264=VERTEX_POINT('',#12047);
#3265=VERTEX_POINT('',#12049);
#3266=VERTEX_POINT('',#12053);
#3267=VERTEX_POINT('',#12054);
#3268=VERTEX_POINT('',#12056);
#3269=VERTEX_POINT('',#12058);
#3270=VERTEX_POINT('',#12065);
#3271=VERTEX_POINT('',#12067);
#3272=VERTEX_POINT('',#12074);
#3273=VERTEX_POINT('',#12076);
#3274=VERTEX_POINT('',#12078);
#3275=VERTEX_POINT('',#12082);
#3276=VERTEX_POINT('',#12084);
#3277=VERTEX_POINT('',#12086);
#3278=VERTEX_POINT('',#12088);
#3279=VERTEX_POINT('',#12090);
#3280=VERTEX_POINT('',#12092);
#3281=VERTEX_POINT('',#12095);
#3282=VERTEX_POINT('',#12097);
#3283=VERTEX_POINT('',#12099);
#3284=VERTEX_POINT('',#12101);
#3285=VERTEX_POINT('',#12104);
#3286=VERTEX_POINT('',#12108);
#3287=VERTEX_POINT('',#12110);
#3288=VERTEX_POINT('',#12112);
#3289=VERTEX_POINT('',#12115);
#3290=VERTEX_POINT('',#12119);
#3291=VERTEX_POINT('',#12121);
#3292=VERTEX_POINT('',#12123);
#3293=VERTEX_POINT('',#12128);
#3294=VERTEX_POINT('',#12131);
#3295=VERTEX_POINT('',#12133);
#3296=VERTEX_POINT('',#12137);
#3297=VERTEX_POINT('',#12140);
#3298=VERTEX_POINT('',#12144);
#3299=VERTEX_POINT('',#12148);
#3300=VERTEX_POINT('',#12152);
#3301=VERTEX_POINT('',#12154);
#3302=VERTEX_POINT('',#12156);
#3303=VERTEX_POINT('',#12158);
#3304=VERTEX_POINT('',#12162);
#3305=VERTEX_POINT('',#12164);
#3306=VERTEX_POINT('',#12168);
#3307=VERTEX_POINT('',#12170);
#3308=VERTEX_POINT('',#12172);
#3309=VERTEX_POINT('',#12176);
#3310=VERTEX_POINT('',#12180);
#3311=VERTEX_POINT('',#12184);
#3312=VERTEX_POINT('',#12185);
#3313=VERTEX_POINT('',#12187);
#3314=VERTEX_POINT('',#12189);
#3315=VERTEX_POINT('',#12192);
#3316=VERTEX_POINT('',#12194);
#3317=VERTEX_POINT('',#12197);
#3318=VERTEX_POINT('',#12200);
#3319=VERTEX_POINT('',#12206);
#3320=VERTEX_POINT('',#12210);
#3321=VERTEX_POINT('',#12216);
#3322=VERTEX_POINT('',#12225);
#3323=VERTEX_POINT('',#12229);
#3324=VERTEX_POINT('',#12237);
#3325=VERTEX_POINT('',#12239);
#3326=VERTEX_POINT('',#12243);
#3327=VERTEX_POINT('',#12247);
#3328=VERTEX_POINT('',#12251);
#3329=VERTEX_POINT('',#12253);
#3330=VERTEX_POINT('',#12257);
#3331=VERTEX_POINT('',#12287);
#3332=VERTEX_POINT('',#12289);
#3333=VERTEX_POINT('',#12293);
#3334=VERTEX_POINT('',#12305);
#3335=VERTEX_POINT('',#12309);
#3336=VERTEX_POINT('',#12313);
#3337=VERTEX_POINT('',#12317);
#3338=VERTEX_POINT('',#12328);
#3339=VERTEX_POINT('',#12330);
#3340=VERTEX_POINT('',#12334);
#3341=VERTEX_POINT('',#12338);
#3342=VERTEX_POINT('',#12342);
#3343=VERTEX_POINT('',#12348);
#3344=VERTEX_POINT('',#12352);
#3345=VERTEX_POINT('',#12354);
#3346=VERTEX_POINT('',#12360);
#3347=VERTEX_POINT('',#12364);
#3348=VERTEX_POINT('',#12368);
#3349=VERTEX_POINT('',#12372);
#3350=VERTEX_POINT('',#12376);
#3351=VERTEX_POINT('',#12380);
#3912=EDGE_CURVE('',#3178,#3179,#2022,.T.);
#3913=EDGE_CURVE('',#3179,#3180,#1950,.T.);
#3914=EDGE_CURVE('',#3180,#3181,#1470,.T.);
#3915=EDGE_CURVE('',#3182,#3181,#2023,.T.);
#3916=EDGE_CURVE('',#3182,#3183,#1471,.F.);
#3917=EDGE_CURVE('',#3183,#3184,#2024,.T.);
#3918=EDGE_CURVE('',#3178,#3184,#1472,.T.);
#3919=EDGE_CURVE('',#3181,#3185,#2025,.T.);
#3920=EDGE_CURVE('',#3185,#3186,#2026,.T.);
#3921=EDGE_CURVE('',#3186,#3182,#2027,.F.);
#3922=EDGE_CURVE('',#3187,#3188,#2028,.T.);
#3923=EDGE_CURVE('',#3189,#3187,#2029,.T.);
#3924=EDGE_CURVE('',#3189,#3179,#2030,.T.);
#3925=EDGE_CURVE('',#3190,#3178,#2031,.T.);
#3926=EDGE_CURVE('',#3188,#3190,#2032,.T.);
#3927=EDGE_CURVE('',#3191,#3189,#1473,.T.);
#3928=EDGE_CURVE('',#3191,#3180,#2033,.T.);
#3929=EDGE_CURVE('',#3192,#3191,#2034,.T.);
#3930=EDGE_CURVE('',#3192,#3193,#2035,.T.);
#3931=EDGE_CURVE('',#3185,#3193,#2036,.T.);
#3932=EDGE_CURVE('',#3194,#3192,#1474,.T.);
#3933=EDGE_CURVE('',#3194,#3195,#2037,.T.);
#3934=EDGE_CURVE('',#3193,#3195,#1475,.T.);
#3935=EDGE_CURVE('',#3196,#3197,#2038,.T.);
#3936=EDGE_CURVE('',#3195,#3196,#2039,.T.);
#3937=EDGE_CURVE('',#3197,#3194,#2040,.T.);
#3938=EDGE_CURVE('',#3198,#3190,#2041,.F.);
#3939=EDGE_CURVE('',#3198,#3199,#2042,.T.);
#3940=EDGE_CURVE('',#3188,#3199,#2043,.T.);
#3941=EDGE_CURVE('',#3200,#3196,#2044,.T.);
#3942=EDGE_CURVE('',#3200,#3201,#2045,.T.);
#3943=EDGE_CURVE('',#3202,#3201,#2046,.F.);
#3944=EDGE_CURVE('',#3203,#3202,#2047,.T.);
#3945=EDGE_CURVE('',#3203,#3186,#2048,.T.);
#3946=EDGE_CURVE('',#3204,#3197,#2049,.T.);
#3947=EDGE_CURVE('',#3205,#3204,#1476,.T.);
#3948=EDGE_CURVE('',#3206,#3205,#2050,.T.);
#3949=EDGE_CURVE('',#3207,#3206,#1477,.T.);
#3950=EDGE_CURVE('',#3208,#3207,#2051,.T.);
#3951=EDGE_CURVE('',#3208,#3209,#2052,.T.);
#3952=EDGE_CURVE('',#3209,#3210,#2053,.T.);
#3953=EDGE_CURVE('',#3210,#3211,#2054,.T.);
#3954=EDGE_CURVE('',#3211,#3212,#1478,.T.);
#3955=EDGE_CURVE('',#3212,#3213,#1479,.T.);
#3956=EDGE_CURVE('',#3213,#3214,#2055,.T.);
#3957=EDGE_CURVE('',#3214,#3215,#1480,.T.);
#3958=EDGE_CURVE('',#3215,#3200,#1481,.T.);
#3959=EDGE_CURVE('',#3216,#3217,#1482,.T.);
#3960=EDGE_CURVE('',#3217,#3218,#2056,.T.);
#3961=EDGE_CURVE('',#3218,#3219,#1483,.F.);
#3962=EDGE_CURVE('',#3219,#3216,#2057,.T.);
#3963=EDGE_CURVE('',#3220,#3221,#2058,.T.);
#3964=EDGE_CURVE('',#3221,#3222,#1484,.T.);
#3965=EDGE_CURVE('',#3222,#3223,#2059,.T.);
#3966=EDGE_CURVE('',#3223,#3220,#237,.T.);
#3967=EDGE_CURVE('',#3223,#3224,#2060,.T.);
#3968=EDGE_CURVE('',#3224,#3225,#238,.T.);
#3969=EDGE_CURVE('',#3225,#3220,#2061,.T.);
#3970=EDGE_CURVE('',#3226,#3216,#1485,.T.);
#3971=EDGE_CURVE('',#3216,#3227,#2062,.T.);
#3972=EDGE_CURVE('',#3227,#3228,#1486,.T.);
#3973=EDGE_CURVE('',#3228,#3226,#2063,.T.);
#3974=EDGE_CURVE('',#3229,#3230,#1487,.T.);
#3975=EDGE_CURVE('',#3230,#3228,#1488,.T.);
#3976=EDGE_CURVE('',#3227,#3229,#1489,.T.);
#3977=EDGE_CURVE('',#3224,#3230,#2064,.T.);
#3978=EDGE_CURVE('',#3229,#3225,#2065,.T.);
#3979=EDGE_CURVE('',#3231,#3232,#1490,.T.);
#3980=EDGE_CURVE('',#3232,#3222,#1491,.T.);
#3981=EDGE_CURVE('',#3221,#3231,#1492,.T.);
#3982=EDGE_CURVE('',#3233,#3234,#1493,.T.);
#3983=EDGE_CURVE('',#3234,#3232,#2066,.T.);
#3984=EDGE_CURVE('',#3231,#3233,#2067,.T.);
#3985=EDGE_CURVE('',#3226,#3217,#1494,.T.);
#3986=EDGE_CURVE('',#3235,#3233,#1495,.T.);
#3987=EDGE_CURVE('',#3233,#3236,#2068,.T.);
#3988=EDGE_CURVE('',#3236,#3237,#1496,.F.);
#3989=EDGE_CURVE('',#3237,#3235,#2069,.T.);
#3990=EDGE_CURVE('',#3235,#3234,#1497,.T.);
#3991=EDGE_CURVE('',#3238,#3218,#2070,.T.);
#3992=EDGE_CURVE('',#3239,#3217,#2071,.T.);
#3993=EDGE_CURVE('',#3240,#3239,#2072,.T.);
#3994=EDGE_CURVE('',#3240,#3241,#2073,.T.);
#3995=EDGE_CURVE('',#3242,#3241,#2074,.T.);
#3996=EDGE_CURVE('',#3243,#3242,#2075,.T.);
#3997=EDGE_CURVE('',#3206,#3243,#2076,.T.);
#3998=EDGE_CURVE('',#3205,#3238,#2077,.T.);
#3999=EDGE_CURVE('',#3226,#3244,#2078,.T.);
#4000=EDGE_CURVE('',#3244,#3239,#1498,.T.);
#4001=EDGE_CURVE('',#3245,#3234,#2079,.T.);
#4002=EDGE_CURVE('',#3246,#3245,#2080,.T.);
#4003=EDGE_CURVE('',#3247,#3246,#1499,.T.);
#4004=EDGE_CURVE('',#3248,#3247,#1500,.T.);
#4005=EDGE_CURVE('',#3249,#3248,#2081,.T.);
#4006=EDGE_CURVE('',#3250,#3249,#1501,.T.);
#4007=EDGE_CURVE('',#3251,#3250,#2082,.T.);
#4008=EDGE_CURVE('',#3252,#3251,#1502,.T.);
#4009=EDGE_CURVE('',#3253,#3252,#2083,.T.);
#4010=EDGE_CURVE('',#3254,#3253,#2084,.T.);
#4011=EDGE_CURVE('',#3255,#3254,#1503,.T.);
#4012=EDGE_CURVE('',#3244,#3255,#2085,.T.);
#4013=EDGE_CURVE('',#3235,#3256,#2086,.T.);
#4014=EDGE_CURVE('',#3256,#3245,#1504,.T.);
#4015=EDGE_CURVE('',#3237,#3257,#2087,.T.);
#4016=EDGE_CURVE('',#3258,#3257,#2088,.T.);
#4017=EDGE_CURVE('',#3258,#3259,#2089,.T.);
#4018=EDGE_CURVE('',#3259,#3260,#2090,.T.);
#4019=EDGE_CURVE('',#3260,#3261,#2091,.T.);
#4020=EDGE_CURVE('',#3256,#3261,#2092,.T.);
#4021=EDGE_CURVE('',#3262,#3263,#2093,.T.);
#4022=EDGE_CURVE('',#3264,#3262,#2094,.T.);
#4023=EDGE_CURVE('',#3265,#3264,#2095,.T.);
#4024=EDGE_CURVE('',#3263,#3265,#2096,.T.);
#4025=EDGE_CURVE('',#3266,#3267,#2097,.T.);
#4026=EDGE_CURVE('',#3268,#3266,#2098,.T.);
#4027=EDGE_CURVE('',#3269,#3268,#2099,.T.);
#4028=EDGE_CURVE('',#3269,#3267,#2100,.T.);
#4029=EDGE_CURVE('',#3267,#3262,#1505,.T.);
#4030=EDGE_CURVE('',#3264,#3269,#1506,.T.);
#4031=EDGE_CURVE('',#3209,#3270,#2101,.T.);
#4032=EDGE_CURVE('',#3271,#3208,#2102,.T.);
#4033=EDGE_CURVE('',#3271,#3270,#2103,.T.);
#4034=EDGE_CURVE('',#3270,#3266,#1507,.T.);
#4035=EDGE_CURVE('',#3268,#3271,#1508,.T.);
#4036=EDGE_CURVE('',#3272,#3207,#2104,.T.);
#4037=EDGE_CURVE('',#3273,#3272,#2105,.T.);
#4038=EDGE_CURVE('',#3274,#3273,#2106,.T.);
#4039=EDGE_CURVE('',#3274,#3265,#2107,.T.);
#4040=EDGE_CURVE('',#3199,#3275,#1509,.T.);
#4041=EDGE_CURVE('',#3275,#3276,#2108,.T.);
#4042=EDGE_CURVE('',#3276,#3277,#1510,.T.);
#4043=EDGE_CURVE('',#3277,#3278,#2109,.T.);
#4044=EDGE_CURVE('',#3278,#3279,#1511,.T.);
#4045=EDGE_CURVE('',#3279,#3280,#2110,.T.);
#4046=EDGE_CURVE('',#3280,#3263,#2111,.T.);
#4047=EDGE_CURVE('',#3281,#3274,#1512,.T.);
#4048=EDGE_CURVE('',#3282,#3281,#2112,.T.);
#4049=EDGE_CURVE('',#3283,#3282,#1513,.T.);
#4050=EDGE_CURVE('',#3284,#3283,#2113,.T.);
#4051=EDGE_CURVE('',#3259,#3284,#1514,.T.);
#4052=EDGE_CURVE('',#3285,#3258,#1515,.T.);
#4053=EDGE_CURVE('',#3187,#3285,#2114,.T.);
#4054=EDGE_CURVE('',#3286,#3286,#1516,.T.);
#4055=EDGE_CURVE('',#3286,#3287,#2115,.T.);
#4056=EDGE_CURVE('',#3288,#3287,#1517,.T.);
#4057=EDGE_CURVE('',#3277,#3288,#2116,.T.);
#4058=EDGE_CURVE('',#3289,#3276,#2117,.T.);
#4059=EDGE_CURVE('',#3287,#3289,#1518,.T.);
#4060=EDGE_CURVE('',#3290,#3290,#1519,.T.);
#4061=EDGE_CURVE('',#3290,#3291,#2118,.T.);
#4062=EDGE_CURVE('',#3292,#3291,#1520,.T.);
#4063=EDGE_CURVE('',#3275,#3292,#2119,.T.);
#4064=EDGE_CURVE('',#3291,#3198,#1521,.T.);
#4065=EDGE_CURVE('',#3293,#3293,#1522,.T.);
#4066=EDGE_CURVE('',#3293,#3212,#2120,.T.);
#4067=EDGE_CURVE('',#3294,#3211,#2121,.T.);
#4068=EDGE_CURVE('',#3295,#3294,#1523,.T.);
#4069=EDGE_CURVE('',#3213,#3295,#2122,.T.);
#4070=EDGE_CURVE('',#3296,#3296,#1524,.T.);
#4071=EDGE_CURVE('',#3296,#3215,#2123,.T.);
#4072=EDGE_CURVE('',#3297,#3214,#2124,.T.);
#4073=EDGE_CURVE('',#3201,#3297,#1525,.T.);
#4074=EDGE_CURVE('',#3288,#3298,#2125,.T.);
#4075=EDGE_CURVE('',#3278,#3298,#2126,.T.);
#4076=EDGE_CURVE('',#3184,#3299,#2127,.T.);
#4077=EDGE_CURVE('',#3299,#3292,#2128,.T.);
#4078=EDGE_CURVE('',#3294,#3300,#2129,.T.);
#4079=EDGE_CURVE('',#3300,#3301,#2130,.T.);
#4080=EDGE_CURVE('',#3301,#3302,#1526,.T.);
#4081=EDGE_CURVE('',#3302,#3303,#2131,.T.);
#4082=EDGE_CURVE('',#3303,#3295,#2132,.T.);
#4083=EDGE_CURVE('',#3210,#3304,#2133,.T.);
#4084=EDGE_CURVE('',#3305,#3304,#2134,.T.);
#4085=EDGE_CURVE('',#3300,#3305,#2135,.T.);
#4086=EDGE_CURVE('',#3303,#3306,#2136,.T.);
#4087=EDGE_CURVE('',#3307,#3306,#2137,.T.);
#4088=EDGE_CURVE('',#3308,#3307,#2138,.F.);
#4089=EDGE_CURVE('',#3297,#3308,#2139,.T.);
#4090=EDGE_CURVE('',#3309,#3305,#2140,.T.);
#4091=EDGE_CURVE('',#3309,#3301,#2141,.T.);
#4092=EDGE_CURVE('',#3280,#3310,#2142,.T.);
#4093=EDGE_CURVE('',#3304,#3310,#2143,.T.);
#4094=EDGE_CURVE('',#3311,#3312,#1527,.T.);
#4095=EDGE_CURVE('',#3312,#3313,#2144,.T.);
#4096=EDGE_CURVE('',#3313,#3314,#2145,.T.);
#4097=EDGE_CURVE('',#3183,#3314,#2146,.F.);
#4098=EDGE_CURVE('',#3315,#3203,#2147,.F.);
#4099=EDGE_CURVE('',#3316,#3315,#1528,.F.);
#4100=EDGE_CURVE('',#3307,#3316,#2148,.F.);
#4101=EDGE_CURVE('',#3306,#3317,#2149,.T.);
#4102=EDGE_CURVE('',#3317,#3309,#1529,.T.);
#4103=EDGE_CURVE('',#3310,#3318,#2150,.T.);
#4104=EDGE_CURVE('',#3318,#3311,#1530,.T.);
#4105=EDGE_CURVE('',#3279,#3318,#2151,.T.);
#4106=EDGE_CURVE('',#3298,#3319,#1531,.F.);
#4107=EDGE_CURVE('',#3319,#3311,#2152,.T.);
#4108=EDGE_CURVE('',#3320,#3319,#1532,.T.);
#4109=EDGE_CURVE('',#3312,#3320,#2153,.T.);
#4110=EDGE_CURVE('',#3317,#3302,#2154,.T.);
#4111=EDGE_CURVE('',#3321,#3320,#2155,.T.);
#4112=EDGE_CURVE('',#3321,#3313,#2156,.T.);
#4113=EDGE_CURVE('',#3289,#3321,#2157,.T.);
#4114=EDGE_CURVE('',#3314,#3299,#2158,.F.);
#4115=EDGE_CURVE('',#3316,#3322,#2159,.T.);
#4116=EDGE_CURVE('',#3308,#3322,#2160,.T.);
#4117=EDGE_CURVE('',#3323,#3202,#2161,.T.);
#4118=EDGE_CURVE('',#3315,#3323,#2162,.T.);
#4119=EDGE_CURVE('',#3322,#3323,#1533,.T.);
#4120=EDGE_CURVE('',#3253,#3324,#1534,.T.);
#4121=EDGE_CURVE('',#3324,#3325,#2163,.T.);
#4122=EDGE_CURVE('',#3325,#3254,#1535,.T.);
#4123=EDGE_CURVE('',#3326,#3255,#1536,.T.);
#4124=EDGE_CURVE('',#3325,#3326,#1537,.T.);
#4125=EDGE_CURVE('',#3327,#3244,#1538,.T.);
#4126=EDGE_CURVE('',#3326,#3327,#2164,.T.);
#4127=EDGE_CURVE('',#3247,#3328,#1539,.T.);
#4128=EDGE_CURVE('',#3328,#3329,#1540,.T.);
#4129=EDGE_CURVE('',#3329,#3248,#1541,.T.);
#4130=EDGE_CURVE('',#3330,#3249,#1542,.T.);
#4131=EDGE_CURVE('',#3329,#3330,#2165,.T.);
#4132=EDGE_CURVE('',#3273,#3250,#1543,.T.);
#4133=EDGE_CURVE('',#3330,#3273,#1544,.T.);
#4134=EDGE_CURVE('',#3272,#3251,#1545,.T.);
#4135=EDGE_CURVE('',#3243,#3252,#1546,.T.);
#4136=EDGE_CURVE('',#3272,#3243,#1547,.T.);
#4137=EDGE_CURVE('',#3242,#3253,#1548,.T.);
#4138=EDGE_CURVE('',#3245,#3331,#1549,.T.);
#4139=EDGE_CURVE('',#3331,#3332,#2166,.T.);
#4140=EDGE_CURVE('',#3332,#3246,#1550,.T.);
#4141=EDGE_CURVE('',#3333,#3247,#1551,.T.);
#4142=EDGE_CURVE('',#3332,#3333,#1552,.T.);
#4143=EDGE_CURVE('',#3256,#3331,#1553,.T.);
#4144=EDGE_CURVE('',#3333,#3328,#1554,.T.);
#4145=EDGE_CURVE('',#3242,#3324,#1555,.T.);
#4146=EDGE_CURVE('',#3327,#3239,#1556,.T.);
#4147=EDGE_CURVE('',#3327,#3334,#2167,.T.);
#4148=EDGE_CURVE('',#3334,#3240,#1557,.F.);
#4149=EDGE_CURVE('',#3326,#3335,#2168,.T.);
#4150=EDGE_CURVE('',#3335,#3334,#2169,.T.);
#4151=EDGE_CURVE('',#3325,#3336,#2170,.T.);
#4152=EDGE_CURVE('',#3336,#3335,#1558,.T.);
#4153=EDGE_CURVE('',#3337,#3324,#2171,.T.);
#4154=EDGE_CURVE('',#3337,#3336,#2172,.T.);
#4155=EDGE_CURVE('',#3241,#3337,#1559,.F.);
#4156=EDGE_CURVE('',#3330,#3281,#2173,.T.);
#4157=EDGE_CURVE('',#3282,#3329,#2174,.T.);
#4158=EDGE_CURVE('',#3338,#3328,#2175,.T.);
#4159=EDGE_CURVE('',#3339,#3338,#1560,.T.);
#4160=EDGE_CURVE('',#3283,#3339,#2176,.T.);
#4161=EDGE_CURVE('',#3333,#3340,#2177,.T.);
#4162=EDGE_CURVE('',#3338,#3340,#1561,.T.);
#4163=EDGE_CURVE('',#3332,#3341,#2178,.T.);
#4164=EDGE_CURVE('',#3341,#3340,#1562,.T.);
#4165=EDGE_CURVE('',#3342,#3331,#2179,.T.);
#4166=EDGE_CURVE('',#3342,#3341,#2180,.T.);
#4167=EDGE_CURVE('',#3261,#3342,#1563,.F.);
#4168=EDGE_CURVE('',#3219,#3343,#2181,.T.);
#4169=EDGE_CURVE('',#3227,#3343,#2182,.T.);
#4170=EDGE_CURVE('',#3229,#3344,#2183,.T.);
#4171=EDGE_CURVE('',#3344,#3345,#2184,.T.);
#4172=EDGE_CURVE('',#3225,#3345,#2185,.T.);
#4173=EDGE_CURVE('',#3343,#3344,#1564,.T.);
#4174=EDGE_CURVE('',#3346,#3238,#1565,.T.);
#4175=EDGE_CURVE('',#3345,#3346,#2186,.T.);
#4176=EDGE_CURVE('',#3347,#3339,#2187,.T.);
#4177=EDGE_CURVE('',#3347,#3260,#1566,.T.);
#4178=EDGE_CURVE('',#3231,#3348,#2188,.T.);
#4179=EDGE_CURVE('',#3348,#3236,#2189,.T.);
#4180=EDGE_CURVE('',#3221,#3349,#2190,.T.);
#4181=EDGE_CURVE('',#3349,#3348,#1567,.T.);
#4182=EDGE_CURVE('',#3350,#3220,#2191,.T.);
#4183=EDGE_CURVE('',#3350,#3349,#2192,.T.);
#4184=EDGE_CURVE('',#3351,#3350,#2193,.T.);
#4185=EDGE_CURVE('',#3257,#3351,#1568,.T.);
#4186=EDGE_CURVE('',#3284,#3347,#2194,.T.);
#4187=EDGE_CURVE('',#3285,#3351,#2195,.T.);
#4188=EDGE_CURVE('',#3204,#3346,#2196,.T.);
#5089=ORIENTED_EDGE('',*,*,#3912,.T.);
#5090=ORIENTED_EDGE('',*,*,#3913,.T.);
#5091=ORIENTED_EDGE('',*,*,#3914,.T.);
#5092=ORIENTED_EDGE('',*,*,#3915,.F.);
#5093=ORIENTED_EDGE('',*,*,#3916,.T.);
#5094=ORIENTED_EDGE('',*,*,#3917,.T.);
#5095=ORIENTED_EDGE('',*,*,#3918,.F.);
#5096=ORIENTED_EDGE('',*,*,#3919,.T.);
#5097=ORIENTED_EDGE('',*,*,#3920,.T.);
#5098=ORIENTED_EDGE('',*,*,#3921,.T.);
#5099=ORIENTED_EDGE('',*,*,#3915,.T.);
#5100=ORIENTED_EDGE('',*,*,#3922,.F.);
#5101=ORIENTED_EDGE('',*,*,#3923,.F.);
#5102=ORIENTED_EDGE('',*,*,#3924,.T.);
#5103=ORIENTED_EDGE('',*,*,#3912,.F.);
#5104=ORIENTED_EDGE('',*,*,#3925,.F.);
#5105=ORIENTED_EDGE('',*,*,#3926,.F.);
#5106=ORIENTED_EDGE('',*,*,#3927,.F.);
#5107=ORIENTED_EDGE('',*,*,#3928,.T.);
#5108=ORIENTED_EDGE('',*,*,#3913,.F.);
#5109=ORIENTED_EDGE('',*,*,#3924,.F.);
#5110=ORIENTED_EDGE('',*,*,#3929,.F.);
#5111=ORIENTED_EDGE('',*,*,#3930,.T.);
#5112=ORIENTED_EDGE('',*,*,#3931,.F.);
#5113=ORIENTED_EDGE('',*,*,#3919,.F.);
#5114=ORIENTED_EDGE('',*,*,#3914,.F.);
#5115=ORIENTED_EDGE('',*,*,#3928,.F.);
#5116=ORIENTED_EDGE('',*,*,#3932,.F.);
#5117=ORIENTED_EDGE('',*,*,#3933,.T.);
#5118=ORIENTED_EDGE('',*,*,#3934,.F.);
#5119=ORIENTED_EDGE('',*,*,#3930,.F.);
#5120=ORIENTED_EDGE('',*,*,#3935,.F.);
#5121=ORIENTED_EDGE('',*,*,#3936,.F.);
#5122=ORIENTED_EDGE('',*,*,#3933,.F.);
#5123=ORIENTED_EDGE('',*,*,#3937,.F.);
#5124=ORIENTED_EDGE('',*,*,#3926,.T.);
#5125=ORIENTED_EDGE('',*,*,#3938,.F.);
#5126=ORIENTED_EDGE('',*,*,#3939,.T.);
#5127=ORIENTED_EDGE('',*,*,#3940,.F.);
#5128=ORIENTED_EDGE('',*,*,#3931,.T.);
#5129=ORIENTED_EDGE('',*,*,#3934,.T.);
#5130=ORIENTED_EDGE('',*,*,#3936,.T.);
#5131=ORIENTED_EDGE('',*,*,#3941,.F.);
#5132=ORIENTED_EDGE('',*,*,#3942,.T.);
#5133=ORIENTED_EDGE('',*,*,#3943,.F.);
#5134=ORIENTED_EDGE('',*,*,#3944,.F.);
#5135=ORIENTED_EDGE('',*,*,#3945,.T.);
#5136=ORIENTED_EDGE('',*,*,#3920,.F.);
#5137=ORIENTED_EDGE('',*,*,#3935,.T.);
#5138=ORIENTED_EDGE('',*,*,#3946,.F.);
#5139=ORIENTED_EDGE('',*,*,#3947,.F.);
#5140=ORIENTED_EDGE('',*,*,#3948,.F.);
#5141=ORIENTED_EDGE('',*,*,#3949,.F.);
#5142=ORIENTED_EDGE('',*,*,#3950,.F.);
#5143=ORIENTED_EDGE('',*,*,#3951,.T.);
#5144=ORIENTED_EDGE('',*,*,#3952,.T.);
#5145=ORIENTED_EDGE('',*,*,#3953,.T.);
#5146=ORIENTED_EDGE('',*,*,#3954,.T.);
#5147=ORIENTED_EDGE('',*,*,#3955,.T.);
#5148=ORIENTED_EDGE('',*,*,#3956,.T.);
#5149=ORIENTED_EDGE('',*,*,#3957,.T.);
#5150=ORIENTED_EDGE('',*,*,#3958,.T.);
#5151=ORIENTED_EDGE('',*,*,#3941,.T.);
#5152=ORIENTED_EDGE('',*,*,#3959,.T.);
#5153=ORIENTED_EDGE('',*,*,#3960,.T.);
#5154=ORIENTED_EDGE('',*,*,#3961,.T.);
#5155=ORIENTED_EDGE('',*,*,#3962,.T.);
#5156=ORIENTED_EDGE('',*,*,#3963,.T.);
#5157=ORIENTED_EDGE('',*,*,#3964,.T.);
#5158=ORIENTED_EDGE('',*,*,#3965,.T.);
#5159=ORIENTED_EDGE('',*,*,#3966,.T.);
#5160=ORIENTED_EDGE('',*,*,#3967,.T.);
#5161=ORIENTED_EDGE('',*,*,#3968,.T.);
#5162=ORIENTED_EDGE('',*,*,#3969,.T.);
#5163=ORIENTED_EDGE('',*,*,#3966,.F.);
#5164=ORIENTED_EDGE('',*,*,#3970,.T.);
#5165=ORIENTED_EDGE('',*,*,#3971,.T.);
#5166=ORIENTED_EDGE('',*,*,#3972,.T.);
#5167=ORIENTED_EDGE('',*,*,#3973,.T.);
#5168=ORIENTED_EDGE('',*,*,#3974,.T.);
#5169=ORIENTED_EDGE('',*,*,#3975,.T.);
#5170=ORIENTED_EDGE('',*,*,#3972,.F.);
#5171=ORIENTED_EDGE('',*,*,#3976,.T.);
#5172=ORIENTED_EDGE('',*,*,#3977,.T.);
#5173=ORIENTED_EDGE('',*,*,#3974,.F.);
#5174=ORIENTED_EDGE('',*,*,#3978,.T.);
#5175=ORIENTED_EDGE('',*,*,#3968,.F.);
#5176=ORIENTED_EDGE('',*,*,#3979,.T.);
#5177=ORIENTED_EDGE('',*,*,#3980,.T.);
#5178=ORIENTED_EDGE('',*,*,#3964,.F.);
#5179=ORIENTED_EDGE('',*,*,#3981,.T.);
#5180=ORIENTED_EDGE('',*,*,#3982,.T.);
#5181=ORIENTED_EDGE('',*,*,#3983,.T.);
#5182=ORIENTED_EDGE('',*,*,#3979,.F.);
#5183=ORIENTED_EDGE('',*,*,#3984,.T.);
#5184=ORIENTED_EDGE('',*,*,#3970,.F.);
#5185=ORIENTED_EDGE('',*,*,#3985,.T.);
#5186=ORIENTED_EDGE('',*,*,#3959,.F.);
#5187=ORIENTED_EDGE('',*,*,#3986,.T.);
#5188=ORIENTED_EDGE('',*,*,#3987,.T.);
#5189=ORIENTED_EDGE('',*,*,#3988,.T.);
#5190=ORIENTED_EDGE('',*,*,#3989,.T.);
#5191=ORIENTED_EDGE('',*,*,#3986,.F.);
#5192=ORIENTED_EDGE('',*,*,#3990,.T.);
#5193=ORIENTED_EDGE('',*,*,#3982,.F.);
#5194=ORIENTED_EDGE('',*,*,#3991,.T.);
#5195=ORIENTED_EDGE('',*,*,#3960,.F.);
#5196=ORIENTED_EDGE('',*,*,#3992,.F.);
#5197=ORIENTED_EDGE('',*,*,#3993,.F.);
#5198=ORIENTED_EDGE('',*,*,#3994,.T.);
#5199=ORIENTED_EDGE('',*,*,#3995,.F.);
#5200=ORIENTED_EDGE('',*,*,#3996,.F.);
#5201=ORIENTED_EDGE('',*,*,#3997,.F.);
#5202=ORIENTED_EDGE('',*,*,#3948,.T.);
#5203=ORIENTED_EDGE('',*,*,#3998,.T.);
#5204=ORIENTED_EDGE('',*,*,#3985,.F.);
#5205=ORIENTED_EDGE('',*,*,#3999,.T.);
#5206=ORIENTED_EDGE('',*,*,#4000,.T.);
#5207=ORIENTED_EDGE('',*,*,#3992,.T.);
#5208=ORIENTED_EDGE('',*,*,#3973,.F.);
#5209=ORIENTED_EDGE('',*,*,#3975,.F.);
#5210=ORIENTED_EDGE('',*,*,#3977,.F.);
#5211=ORIENTED_EDGE('',*,*,#3967,.F.);
#5212=ORIENTED_EDGE('',*,*,#3965,.F.);
#5213=ORIENTED_EDGE('',*,*,#3980,.F.);
#5214=ORIENTED_EDGE('',*,*,#3983,.F.);
#5215=ORIENTED_EDGE('',*,*,#4001,.F.);
#5216=ORIENTED_EDGE('',*,*,#4002,.F.);
#5217=ORIENTED_EDGE('',*,*,#4003,.F.);
#5218=ORIENTED_EDGE('',*,*,#4004,.F.);
#5219=ORIENTED_EDGE('',*,*,#4005,.F.);
#5220=ORIENTED_EDGE('',*,*,#4006,.F.);
#5221=ORIENTED_EDGE('',*,*,#4007,.F.);
#5222=ORIENTED_EDGE('',*,*,#4008,.F.);
#5223=ORIENTED_EDGE('',*,*,#4009,.F.);
#5224=ORIENTED_EDGE('',*,*,#4010,.F.);
#5225=ORIENTED_EDGE('',*,*,#4011,.F.);
#5226=ORIENTED_EDGE('',*,*,#4012,.F.);
#5227=ORIENTED_EDGE('',*,*,#3999,.F.);
#5228=ORIENTED_EDGE('',*,*,#3990,.F.);
#5229=ORIENTED_EDGE('',*,*,#4013,.T.);
#5230=ORIENTED_EDGE('',*,*,#4014,.T.);
#5231=ORIENTED_EDGE('',*,*,#4001,.T.);
#5232=ORIENTED_EDGE('',*,*,#3989,.F.);
#5233=ORIENTED_EDGE('',*,*,#4015,.T.);
#5234=ORIENTED_EDGE('',*,*,#4016,.F.);
#5235=ORIENTED_EDGE('',*,*,#4017,.T.);
#5236=ORIENTED_EDGE('',*,*,#4018,.T.);
#5237=ORIENTED_EDGE('',*,*,#4019,.T.);
#5238=ORIENTED_EDGE('',*,*,#4020,.F.);
#5239=ORIENTED_EDGE('',*,*,#4013,.F.);
#5240=ORIENTED_EDGE('',*,*,#4021,.F.);
#5241=ORIENTED_EDGE('',*,*,#4022,.F.);
#5242=ORIENTED_EDGE('',*,*,#4023,.F.);
#5243=ORIENTED_EDGE('',*,*,#4024,.F.);
#5244=ORIENTED_EDGE('',*,*,#4025,.F.);
#5245=ORIENTED_EDGE('',*,*,#4026,.F.);
#5246=ORIENTED_EDGE('',*,*,#4027,.F.);
#5247=ORIENTED_EDGE('',*,*,#4028,.T.);
#5248=ORIENTED_EDGE('',*,*,#4029,.F.);
#5249=ORIENTED_EDGE('',*,*,#4028,.F.);
#5250=ORIENTED_EDGE('',*,*,#4030,.F.);
#5251=ORIENTED_EDGE('',*,*,#4022,.T.);
#5252=ORIENTED_EDGE('',*,*,#4031,.F.);
#5253=ORIENTED_EDGE('',*,*,#3951,.F.);
#5254=ORIENTED_EDGE('',*,*,#4032,.F.);
#5255=ORIENTED_EDGE('',*,*,#4033,.T.);
#5256=ORIENTED_EDGE('',*,*,#4034,.F.);
#5257=ORIENTED_EDGE('',*,*,#4033,.F.);
#5258=ORIENTED_EDGE('',*,*,#4035,.F.);
#5259=ORIENTED_EDGE('',*,*,#4026,.T.);
#5260=ORIENTED_EDGE('',*,*,#4023,.T.);
#5261=ORIENTED_EDGE('',*,*,#4030,.T.);
#5262=ORIENTED_EDGE('',*,*,#4027,.T.);
#5263=ORIENTED_EDGE('',*,*,#4035,.T.);
#5264=ORIENTED_EDGE('',*,*,#4032,.T.);
#5265=ORIENTED_EDGE('',*,*,#3950,.T.);
#5266=ORIENTED_EDGE('',*,*,#4036,.F.);
#5267=ORIENTED_EDGE('',*,*,#4037,.F.);
#5268=ORIENTED_EDGE('',*,*,#4038,.F.);
#5269=ORIENTED_EDGE('',*,*,#4039,.T.);
#5270=ORIENTED_EDGE('',*,*,#3922,.T.);
#5271=ORIENTED_EDGE('',*,*,#3940,.T.);
#5272=ORIENTED_EDGE('',*,*,#4040,.T.);
#5273=ORIENTED_EDGE('',*,*,#4041,.T.);
#5274=ORIENTED_EDGE('',*,*,#4042,.T.);
#5275=ORIENTED_EDGE('',*,*,#4043,.T.);
#5276=ORIENTED_EDGE('',*,*,#4044,.T.);
#5277=ORIENTED_EDGE('',*,*,#4045,.T.);
#5278=ORIENTED_EDGE('',*,*,#4046,.T.);
#5279=ORIENTED_EDGE('',*,*,#4024,.T.);
#5280=ORIENTED_EDGE('',*,*,#4039,.F.);
#5281=ORIENTED_EDGE('',*,*,#4047,.F.);
#5282=ORIENTED_EDGE('',*,*,#4048,.F.);
#5283=ORIENTED_EDGE('',*,*,#4049,.F.);
#5284=ORIENTED_EDGE('',*,*,#4050,.F.);
#5285=ORIENTED_EDGE('',*,*,#4051,.F.);
#5286=ORIENTED_EDGE('',*,*,#4017,.F.);
#5287=ORIENTED_EDGE('',*,*,#4052,.F.);
#5288=ORIENTED_EDGE('',*,*,#4053,.F.);
#5289=ORIENTED_EDGE('',*,*,#4054,.F.);
#5290=ORIENTED_EDGE('',*,*,#4055,.T.);
#5291=ORIENTED_EDGE('',*,*,#4056,.F.);
#5292=ORIENTED_EDGE('',*,*,#4057,.F.);
#5293=ORIENTED_EDGE('',*,*,#4042,.F.);
#5294=ORIENTED_EDGE('',*,*,#4058,.F.);
#5295=ORIENTED_EDGE('',*,*,#4059,.F.);
#5296=ORIENTED_EDGE('',*,*,#4055,.F.);
#5297=ORIENTED_EDGE('',*,*,#4060,.F.);
#5298=ORIENTED_EDGE('',*,*,#4061,.T.);
#5299=ORIENTED_EDGE('',*,*,#4062,.F.);
#5300=ORIENTED_EDGE('',*,*,#4063,.F.);
#5301=ORIENTED_EDGE('',*,*,#4040,.F.);
#5302=ORIENTED_EDGE('',*,*,#3939,.F.);
#5303=ORIENTED_EDGE('',*,*,#4064,.F.);
#5304=ORIENTED_EDGE('',*,*,#4061,.F.);
#5305=ORIENTED_EDGE('',*,*,#4065,.F.);
#5306=ORIENTED_EDGE('',*,*,#4066,.T.);
#5307=ORIENTED_EDGE('',*,*,#3954,.F.);
#5308=ORIENTED_EDGE('',*,*,#4067,.F.);
#5309=ORIENTED_EDGE('',*,*,#4068,.F.);
#5310=ORIENTED_EDGE('',*,*,#4069,.F.);
#5311=ORIENTED_EDGE('',*,*,#3955,.F.);
#5312=ORIENTED_EDGE('',*,*,#4066,.F.);
#5313=ORIENTED_EDGE('',*,*,#4070,.F.);
#5314=ORIENTED_EDGE('',*,*,#4071,.T.);
#5315=ORIENTED_EDGE('',*,*,#3957,.F.);
#5316=ORIENTED_EDGE('',*,*,#4072,.F.);
#5317=ORIENTED_EDGE('',*,*,#4073,.F.);
#5318=ORIENTED_EDGE('',*,*,#3942,.F.);
#5319=ORIENTED_EDGE('',*,*,#3958,.F.);
#5320=ORIENTED_EDGE('',*,*,#4071,.F.);
#5321=ORIENTED_EDGE('',*,*,#4057,.T.);
#5322=ORIENTED_EDGE('',*,*,#4074,.T.);
#5323=ORIENTED_EDGE('',*,*,#4075,.F.);
#5324=ORIENTED_EDGE('',*,*,#4043,.F.);
#5325=ORIENTED_EDGE('',*,*,#3925,.T.);
#5326=ORIENTED_EDGE('',*,*,#3918,.T.);
#5327=ORIENTED_EDGE('',*,*,#4076,.T.);
#5328=ORIENTED_EDGE('',*,*,#4077,.T.);
#5329=ORIENTED_EDGE('',*,*,#4062,.T.);
#5330=ORIENTED_EDGE('',*,*,#4064,.T.);
#5331=ORIENTED_EDGE('',*,*,#3938,.T.);
#5332=ORIENTED_EDGE('',*,*,#4068,.T.);
#5333=ORIENTED_EDGE('',*,*,#4078,.T.);
#5334=ORIENTED_EDGE('',*,*,#4079,.T.);
#5335=ORIENTED_EDGE('',*,*,#4080,.T.);
#5336=ORIENTED_EDGE('',*,*,#4081,.T.);
#5337=ORIENTED_EDGE('',*,*,#4082,.T.);
#5338=ORIENTED_EDGE('',*,*,#4067,.T.);
#5339=ORIENTED_EDGE('',*,*,#3953,.F.);
#5340=ORIENTED_EDGE('',*,*,#4083,.T.);
#5341=ORIENTED_EDGE('',*,*,#4084,.F.);
#5342=ORIENTED_EDGE('',*,*,#4085,.F.);
#5343=ORIENTED_EDGE('',*,*,#4078,.F.);
#5344=ORIENTED_EDGE('',*,*,#4069,.T.);
#5345=ORIENTED_EDGE('',*,*,#4082,.F.);
#5346=ORIENTED_EDGE('',*,*,#4086,.T.);
#5347=ORIENTED_EDGE('',*,*,#4087,.F.);
#5348=ORIENTED_EDGE('',*,*,#4088,.F.);
#5349=ORIENTED_EDGE('',*,*,#4089,.F.);
#5350=ORIENTED_EDGE('',*,*,#4072,.T.);
#5351=ORIENTED_EDGE('',*,*,#3956,.F.);
#5352=ORIENTED_EDGE('',*,*,#4090,.F.);
#5353=ORIENTED_EDGE('',*,*,#4091,.T.);
#5354=ORIENTED_EDGE('',*,*,#4079,.F.);
#5355=ORIENTED_EDGE('',*,*,#4085,.T.);
#5356=ORIENTED_EDGE('',*,*,#4021,.T.);
#5357=ORIENTED_EDGE('',*,*,#4046,.F.);
#5358=ORIENTED_EDGE('',*,*,#4092,.T.);
#5359=ORIENTED_EDGE('',*,*,#4093,.F.);
#5360=ORIENTED_EDGE('',*,*,#4083,.F.);
#5361=ORIENTED_EDGE('',*,*,#3952,.F.);
#5362=ORIENTED_EDGE('',*,*,#4031,.T.);
#5363=ORIENTED_EDGE('',*,*,#4034,.T.);
#5364=ORIENTED_EDGE('',*,*,#4025,.T.);
#5365=ORIENTED_EDGE('',*,*,#4029,.T.);
#5366=ORIENTED_EDGE('',*,*,#4094,.T.);
#5367=ORIENTED_EDGE('',*,*,#4095,.T.);
#5368=ORIENTED_EDGE('',*,*,#4096,.T.);
#5369=ORIENTED_EDGE('',*,*,#4097,.F.);
#5370=ORIENTED_EDGE('',*,*,#3916,.F.);
#5371=ORIENTED_EDGE('',*,*,#3921,.F.);
#5372=ORIENTED_EDGE('',*,*,#3945,.F.);
#5373=ORIENTED_EDGE('',*,*,#4098,.F.);
#5374=ORIENTED_EDGE('',*,*,#4099,.F.);
#5375=ORIENTED_EDGE('',*,*,#4100,.F.);
#5376=ORIENTED_EDGE('',*,*,#4087,.T.);
#5377=ORIENTED_EDGE('',*,*,#4101,.T.);
#5378=ORIENTED_EDGE('',*,*,#4102,.T.);
#5379=ORIENTED_EDGE('',*,*,#4090,.T.);
#5380=ORIENTED_EDGE('',*,*,#4084,.T.);
#5381=ORIENTED_EDGE('',*,*,#4093,.T.);
#5382=ORIENTED_EDGE('',*,*,#4103,.T.);
#5383=ORIENTED_EDGE('',*,*,#4104,.T.);
#5384=ORIENTED_EDGE('',*,*,#4103,.F.);
#5385=ORIENTED_EDGE('',*,*,#4092,.F.);
#5386=ORIENTED_EDGE('',*,*,#4045,.F.);
#5387=ORIENTED_EDGE('',*,*,#4105,.T.);
#5388=ORIENTED_EDGE('',*,*,#4104,.F.);
#5389=ORIENTED_EDGE('',*,*,#4105,.F.);
#5390=ORIENTED_EDGE('',*,*,#4044,.F.);
#5391=ORIENTED_EDGE('',*,*,#4075,.T.);
#5392=ORIENTED_EDGE('',*,*,#4106,.T.);
#5393=ORIENTED_EDGE('',*,*,#4107,.T.);
#5394=ORIENTED_EDGE('',*,*,#4094,.F.);
#5395=ORIENTED_EDGE('',*,*,#4107,.F.);
#5396=ORIENTED_EDGE('',*,*,#4108,.F.);
#5397=ORIENTED_EDGE('',*,*,#4109,.F.);
#5398=ORIENTED_EDGE('',*,*,#4101,.F.);
#5399=ORIENTED_EDGE('',*,*,#4086,.F.);
#5400=ORIENTED_EDGE('',*,*,#4081,.F.);
#5401=ORIENTED_EDGE('',*,*,#4110,.F.);
#5402=ORIENTED_EDGE('',*,*,#4095,.F.);
#5403=ORIENTED_EDGE('',*,*,#4109,.T.);
#5404=ORIENTED_EDGE('',*,*,#4111,.F.);
#5405=ORIENTED_EDGE('',*,*,#4112,.T.);
#5406=ORIENTED_EDGE('',*,*,#4056,.T.);
#5407=ORIENTED_EDGE('',*,*,#4059,.T.);
#5408=ORIENTED_EDGE('',*,*,#4113,.T.);
#5409=ORIENTED_EDGE('',*,*,#4111,.T.);
#5410=ORIENTED_EDGE('',*,*,#4108,.T.);
#5411=ORIENTED_EDGE('',*,*,#4106,.F.);
#5412=ORIENTED_EDGE('',*,*,#4074,.F.);
#5413=ORIENTED_EDGE('',*,*,#4058,.T.);
#5414=ORIENTED_EDGE('',*,*,#4041,.F.);
#5415=ORIENTED_EDGE('',*,*,#4063,.T.);
#5416=ORIENTED_EDGE('',*,*,#4077,.F.);
#5417=ORIENTED_EDGE('',*,*,#4114,.F.);
#5418=ORIENTED_EDGE('',*,*,#4096,.F.);
#5419=ORIENTED_EDGE('',*,*,#4112,.F.);
#5420=ORIENTED_EDGE('',*,*,#4113,.F.);
#5421=ORIENTED_EDGE('',*,*,#4102,.F.);
#5422=ORIENTED_EDGE('',*,*,#4110,.T.);
#5423=ORIENTED_EDGE('',*,*,#4080,.F.);
#5424=ORIENTED_EDGE('',*,*,#4091,.F.);
#5425=ORIENTED_EDGE('',*,*,#4088,.T.);
#5426=ORIENTED_EDGE('',*,*,#4100,.T.);
#5427=ORIENTED_EDGE('',*,*,#4115,.T.);
#5428=ORIENTED_EDGE('',*,*,#4116,.F.);
#5429=ORIENTED_EDGE('',*,*,#4098,.T.);
#5430=ORIENTED_EDGE('',*,*,#3944,.T.);
#5431=ORIENTED_EDGE('',*,*,#4117,.F.);
#5432=ORIENTED_EDGE('',*,*,#4118,.F.);
#5433=ORIENTED_EDGE('',*,*,#4099,.T.);
#5434=ORIENTED_EDGE('',*,*,#4118,.T.);
#5435=ORIENTED_EDGE('',*,*,#4119,.F.);
#5436=ORIENTED_EDGE('',*,*,#4115,.F.);
#5437=ORIENTED_EDGE('',*,*,#4073,.T.);
#5438=ORIENTED_EDGE('',*,*,#4089,.T.);
#5439=ORIENTED_EDGE('',*,*,#4116,.T.);
#5440=ORIENTED_EDGE('',*,*,#4119,.T.);
#5441=ORIENTED_EDGE('',*,*,#4117,.T.);
#5442=ORIENTED_EDGE('',*,*,#3943,.T.);
#5443=ORIENTED_EDGE('',*,*,#4097,.T.);
#5444=ORIENTED_EDGE('',*,*,#4114,.T.);
#5445=ORIENTED_EDGE('',*,*,#4076,.F.);
#5446=ORIENTED_EDGE('',*,*,#3917,.F.);
#5447=ORIENTED_EDGE('',*,*,#4120,.T.);
#5448=ORIENTED_EDGE('',*,*,#4121,.T.);
#5449=ORIENTED_EDGE('',*,*,#4122,.T.);
#5450=ORIENTED_EDGE('',*,*,#4010,.T.);
#5451=ORIENTED_EDGE('',*,*,#4123,.T.);
#5452=ORIENTED_EDGE('',*,*,#4011,.T.);
#5453=ORIENTED_EDGE('',*,*,#4122,.F.);
#5454=ORIENTED_EDGE('',*,*,#4124,.T.);
#5455=ORIENTED_EDGE('',*,*,#4125,.T.);
#5456=ORIENTED_EDGE('',*,*,#4012,.T.);
#5457=ORIENTED_EDGE('',*,*,#4123,.F.);
#5458=ORIENTED_EDGE('',*,*,#4126,.T.);
#5459=ORIENTED_EDGE('',*,*,#4127,.T.);
#5460=ORIENTED_EDGE('',*,*,#4128,.T.);
#5461=ORIENTED_EDGE('',*,*,#4129,.T.);
#5462=ORIENTED_EDGE('',*,*,#4004,.T.);
#5463=ORIENTED_EDGE('',*,*,#4130,.T.);
#5464=ORIENTED_EDGE('',*,*,#4005,.T.);
#5465=ORIENTED_EDGE('',*,*,#4129,.F.);
#5466=ORIENTED_EDGE('',*,*,#4131,.T.);
#5467=ORIENTED_EDGE('',*,*,#4132,.T.);
#5468=ORIENTED_EDGE('',*,*,#4006,.T.);
#5469=ORIENTED_EDGE('',*,*,#4130,.F.);
#5470=ORIENTED_EDGE('',*,*,#4133,.T.);
#5471=ORIENTED_EDGE('',*,*,#4134,.T.);
#5472=ORIENTED_EDGE('',*,*,#4007,.T.);
#5473=ORIENTED_EDGE('',*,*,#4132,.F.);
#5474=ORIENTED_EDGE('',*,*,#4037,.T.);
#5475=ORIENTED_EDGE('',*,*,#4135,.T.);
#5476=ORIENTED_EDGE('',*,*,#4008,.T.);
#5477=ORIENTED_EDGE('',*,*,#4134,.F.);
#5478=ORIENTED_EDGE('',*,*,#4136,.T.);
#5479=ORIENTED_EDGE('',*,*,#4137,.T.);
#5480=ORIENTED_EDGE('',*,*,#4009,.T.);
#5481=ORIENTED_EDGE('',*,*,#4135,.F.);
#5482=ORIENTED_EDGE('',*,*,#3996,.T.);
#5483=ORIENTED_EDGE('',*,*,#4138,.T.);
#5484=ORIENTED_EDGE('',*,*,#4139,.T.);
#5485=ORIENTED_EDGE('',*,*,#4140,.T.);
#5486=ORIENTED_EDGE('',*,*,#4002,.T.);
#5487=ORIENTED_EDGE('',*,*,#4141,.T.);
#5488=ORIENTED_EDGE('',*,*,#4003,.T.);
#5489=ORIENTED_EDGE('',*,*,#4140,.F.);
#5490=ORIENTED_EDGE('',*,*,#4142,.T.);
#5491=ORIENTED_EDGE('',*,*,#4014,.F.);
#5492=ORIENTED_EDGE('',*,*,#4143,.T.);
#5493=ORIENTED_EDGE('',*,*,#4138,.F.);
#5494=ORIENTED_EDGE('',*,*,#4141,.F.);
#5495=ORIENTED_EDGE('',*,*,#4144,.T.);
#5496=ORIENTED_EDGE('',*,*,#4127,.F.);
#5497=ORIENTED_EDGE('',*,*,#4137,.F.);
#5498=ORIENTED_EDGE('',*,*,#4145,.T.);
#5499=ORIENTED_EDGE('',*,*,#4120,.F.);
#5500=ORIENTED_EDGE('',*,*,#4125,.F.);
#5501=ORIENTED_EDGE('',*,*,#4146,.T.);
#5502=ORIENTED_EDGE('',*,*,#4000,.F.);
#5503=ORIENTED_EDGE('',*,*,#4146,.F.);
#5504=ORIENTED_EDGE('',*,*,#4147,.T.);
#5505=ORIENTED_EDGE('',*,*,#4148,.T.);
#5506=ORIENTED_EDGE('',*,*,#3993,.T.);
#5507=ORIENTED_EDGE('',*,*,#4126,.F.);
#5508=ORIENTED_EDGE('',*,*,#4149,.T.);
#5509=ORIENTED_EDGE('',*,*,#4150,.T.);
#5510=ORIENTED_EDGE('',*,*,#4147,.F.);
#5511=ORIENTED_EDGE('',*,*,#4124,.F.);
#5512=ORIENTED_EDGE('',*,*,#4151,.T.);
#5513=ORIENTED_EDGE('',*,*,#4152,.T.);
#5514=ORIENTED_EDGE('',*,*,#4149,.F.);
#5515=ORIENTED_EDGE('',*,*,#4121,.F.);
#5516=ORIENTED_EDGE('',*,*,#4153,.F.);
#5517=ORIENTED_EDGE('',*,*,#4154,.T.);
#5518=ORIENTED_EDGE('',*,*,#4151,.F.);
#5519=ORIENTED_EDGE('',*,*,#4145,.F.);
#5520=ORIENTED_EDGE('',*,*,#3995,.T.);
#5521=ORIENTED_EDGE('',*,*,#4155,.T.);
#5522=ORIENTED_EDGE('',*,*,#4153,.T.);
#5523=ORIENTED_EDGE('',*,*,#4136,.F.);
#5524=ORIENTED_EDGE('',*,*,#4036,.T.);
#5525=ORIENTED_EDGE('',*,*,#3949,.T.);
#5526=ORIENTED_EDGE('',*,*,#3997,.T.);
#5527=ORIENTED_EDGE('',*,*,#4133,.F.);
#5528=ORIENTED_EDGE('',*,*,#4156,.T.);
#5529=ORIENTED_EDGE('',*,*,#4047,.T.);
#5530=ORIENTED_EDGE('',*,*,#4038,.T.);
#5531=ORIENTED_EDGE('',*,*,#4131,.F.);
#5532=ORIENTED_EDGE('',*,*,#4157,.F.);
#5533=ORIENTED_EDGE('',*,*,#4048,.T.);
#5534=ORIENTED_EDGE('',*,*,#4156,.F.);
#5535=ORIENTED_EDGE('',*,*,#4128,.F.);
#5536=ORIENTED_EDGE('',*,*,#4158,.F.);
#5537=ORIENTED_EDGE('',*,*,#4159,.F.);
#5538=ORIENTED_EDGE('',*,*,#4160,.F.);
#5539=ORIENTED_EDGE('',*,*,#4049,.T.);
#5540=ORIENTED_EDGE('',*,*,#4157,.T.);
#5541=ORIENTED_EDGE('',*,*,#4144,.F.);
#5542=ORIENTED_EDGE('',*,*,#4161,.T.);
#5543=ORIENTED_EDGE('',*,*,#4162,.F.);
#5544=ORIENTED_EDGE('',*,*,#4158,.T.);
#5545=ORIENTED_EDGE('',*,*,#4142,.F.);
#5546=ORIENTED_EDGE('',*,*,#4163,.T.);
#5547=ORIENTED_EDGE('',*,*,#4164,.T.);
#5548=ORIENTED_EDGE('',*,*,#4161,.F.);
#5549=ORIENTED_EDGE('',*,*,#4139,.F.);
#5550=ORIENTED_EDGE('',*,*,#4165,.F.);
#5551=ORIENTED_EDGE('',*,*,#4166,.T.);
#5552=ORIENTED_EDGE('',*,*,#4163,.F.);
#5553=ORIENTED_EDGE('',*,*,#4143,.F.);
#5554=ORIENTED_EDGE('',*,*,#4020,.T.);
#5555=ORIENTED_EDGE('',*,*,#4167,.T.);
#5556=ORIENTED_EDGE('',*,*,#4165,.T.);
#5557=ORIENTED_EDGE('',*,*,#3962,.F.);
#5558=ORIENTED_EDGE('',*,*,#4168,.T.);
#5559=ORIENTED_EDGE('',*,*,#4169,.F.);
#5560=ORIENTED_EDGE('',*,*,#3971,.F.);
#5561=ORIENTED_EDGE('',*,*,#3978,.F.);
#5562=ORIENTED_EDGE('',*,*,#4170,.T.);
#5563=ORIENTED_EDGE('',*,*,#4171,.T.);
#5564=ORIENTED_EDGE('',*,*,#4172,.F.);
#5565=ORIENTED_EDGE('',*,*,#3976,.F.);
#5566=ORIENTED_EDGE('',*,*,#4169,.T.);
#5567=ORIENTED_EDGE('',*,*,#4173,.T.);
#5568=ORIENTED_EDGE('',*,*,#4170,.F.);
#5569=ORIENTED_EDGE('',*,*,#4173,.F.);
#5570=ORIENTED_EDGE('',*,*,#4168,.F.);
#5571=ORIENTED_EDGE('',*,*,#3961,.F.);
#5572=ORIENTED_EDGE('',*,*,#3991,.F.);
#5573=ORIENTED_EDGE('',*,*,#4174,.F.);
#5574=ORIENTED_EDGE('',*,*,#4175,.F.);
#5575=ORIENTED_EDGE('',*,*,#4171,.F.);
#5576=ORIENTED_EDGE('',*,*,#4070,.T.);
#5577=ORIENTED_EDGE('',*,*,#4176,.T.);
#5578=ORIENTED_EDGE('',*,*,#4159,.T.);
#5579=ORIENTED_EDGE('',*,*,#4162,.T.);
#5580=ORIENTED_EDGE('',*,*,#4164,.F.);
#5581=ORIENTED_EDGE('',*,*,#4166,.F.);
#5582=ORIENTED_EDGE('',*,*,#4167,.F.);
#5583=ORIENTED_EDGE('',*,*,#4019,.F.);
#5584=ORIENTED_EDGE('',*,*,#4177,.F.);
#5585=ORIENTED_EDGE('',*,*,#4054,.T.);
#5586=ORIENTED_EDGE('',*,*,#3984,.F.);
#5587=ORIENTED_EDGE('',*,*,#4178,.T.);
#5588=ORIENTED_EDGE('',*,*,#4179,.T.);
#5589=ORIENTED_EDGE('',*,*,#3987,.F.);
#5590=ORIENTED_EDGE('',*,*,#3981,.F.);
#5591=ORIENTED_EDGE('',*,*,#4180,.T.);
#5592=ORIENTED_EDGE('',*,*,#4181,.T.);
#5593=ORIENTED_EDGE('',*,*,#4178,.F.);
#5594=ORIENTED_EDGE('',*,*,#3963,.F.);
#5595=ORIENTED_EDGE('',*,*,#4182,.F.);
#5596=ORIENTED_EDGE('',*,*,#4183,.T.);
#5597=ORIENTED_EDGE('',*,*,#4180,.F.);
#5598=ORIENTED_EDGE('',*,*,#4183,.F.);
#5599=ORIENTED_EDGE('',*,*,#4184,.F.);
#5600=ORIENTED_EDGE('',*,*,#4185,.F.);
#5601=ORIENTED_EDGE('',*,*,#4015,.F.);
#5602=ORIENTED_EDGE('',*,*,#3988,.F.);
#5603=ORIENTED_EDGE('',*,*,#4179,.F.);
#5604=ORIENTED_EDGE('',*,*,#4181,.F.);
#5605=ORIENTED_EDGE('',*,*,#4060,.T.);
#5606=ORIENTED_EDGE('',*,*,#4152,.F.);
#5607=ORIENTED_EDGE('',*,*,#4154,.F.);
#5608=ORIENTED_EDGE('',*,*,#4155,.F.);
#5609=ORIENTED_EDGE('',*,*,#3994,.F.);
#5610=ORIENTED_EDGE('',*,*,#4148,.F.);
#5611=ORIENTED_EDGE('',*,*,#4150,.F.);
#5612=ORIENTED_EDGE('',*,*,#4065,.T.);
#5613=ORIENTED_EDGE('',*,*,#4176,.F.);
#5614=ORIENTED_EDGE('',*,*,#4186,.F.);
#5615=ORIENTED_EDGE('',*,*,#4050,.T.);
#5616=ORIENTED_EDGE('',*,*,#4160,.T.);
#5617=ORIENTED_EDGE('',*,*,#3923,.T.);
#5618=ORIENTED_EDGE('',*,*,#4053,.T.);
#5619=ORIENTED_EDGE('',*,*,#4187,.T.);
#5620=ORIENTED_EDGE('',*,*,#4184,.T.);
#5621=ORIENTED_EDGE('',*,*,#4182,.T.);
#5622=ORIENTED_EDGE('',*,*,#3969,.F.);
#5623=ORIENTED_EDGE('',*,*,#4172,.T.);
#5624=ORIENTED_EDGE('',*,*,#4175,.T.);
#5625=ORIENTED_EDGE('',*,*,#4188,.F.);
#5626=ORIENTED_EDGE('',*,*,#3946,.T.);
#5627=ORIENTED_EDGE('',*,*,#3937,.T.);
#5628=ORIENTED_EDGE('',*,*,#3932,.T.);
#5629=ORIENTED_EDGE('',*,*,#3929,.T.);
#5630=ORIENTED_EDGE('',*,*,#3927,.T.);
#5631=ORIENTED_EDGE('',*,*,#4177,.T.);
#5632=ORIENTED_EDGE('',*,*,#4018,.F.);
#5633=ORIENTED_EDGE('',*,*,#4051,.T.);
#5634=ORIENTED_EDGE('',*,*,#4186,.T.);
#5635=ORIENTED_EDGE('',*,*,#4185,.T.);
#5636=ORIENTED_EDGE('',*,*,#4187,.F.);
#5637=ORIENTED_EDGE('',*,*,#4052,.T.);
#5638=ORIENTED_EDGE('',*,*,#4016,.T.);
#5639=ORIENTED_EDGE('',*,*,#4174,.T.);
#5640=ORIENTED_EDGE('',*,*,#3998,.F.);
#5641=ORIENTED_EDGE('',*,*,#3947,.T.);
#5642=ORIENTED_EDGE('',*,*,#4188,.T.);
#7443=CYLINDRICAL_SURFACE('',#8262,4.5);
#7444=CYLINDRICAL_SURFACE('',#8268,1.);
#7445=CYLINDRICAL_SURFACE('',#8271,0.999999999999998);
#7446=CYLINDRICAL_SURFACE('',#8284,1.);
#7447=CYLINDRICAL_SURFACE('',#8287,1.);
#7448=CYLINDRICAL_SURFACE('',#8290,1.);
#7449=CYLINDRICAL_SURFACE('',#8292,1.);
#7450=CYLINDRICAL_SURFACE('',#8299,1.);
#7451=CYLINDRICAL_SURFACE('',#8304,1.);
#7452=CYLINDRICAL_SURFACE('',#8308,1.);
#7453=CYLINDRICAL_SURFACE('',#8314,1.);
#7454=CYLINDRICAL_SURFACE('',#8322,1.);
#7455=CYLINDRICAL_SURFACE('',#8327,2.);
#7456=CYLINDRICAL_SURFACE('',#8331,2.);
#7457=CYLINDRICAL_SURFACE('',#8343,1.5);
#7458=CYLINDRICAL_SURFACE('',#8347,1.5);
#7459=CYLINDRICAL_SURFACE('',#8351,1.5);
#7460=CYLINDRICAL_SURFACE('',#8354,1.5);
#7461=CYLINDRICAL_SURFACE('',#8371,3.);
#7462=CYLINDRICAL_SURFACE('',#8373,4.5);
#7463=CYLINDRICAL_SURFACE('',#8379,4.5);
#7464=CYLINDRICAL_SURFACE('',#8382,4.5);
#7465=CYLINDRICAL_SURFACE('',#8386,1.);
#7466=CYLINDRICAL_SURFACE('',#8392,1.);
#7467=CYLINDRICAL_SURFACE('',#8398,1.);
#7468=CYLINDRICAL_SURFACE('',#8402,1.);
#7469=CYLINDRICAL_SURFACE('',#8406,1.);
#7470=CYLINDRICAL_SURFACE('',#8408,1.);
#7471=CYLINDRICAL_SURFACE('',#8422,1.);
#7472=CYLINDRICAL_SURFACE('',#8425,2.5);
#7473=CYLINDRICAL_SURFACE('',#8428,1.);
#7474=CYLINDRICAL_SURFACE('',#8430,2.);
#7475=CYLINDRICAL_SURFACE('',#8431,2.);
#7476=CYLINDRICAL_SURFACE('',#8433,0.999999999999996);
#7477=CYLINDRICAL_SURFACE('',#8435,1.);
#7478=CYLINDRICAL_SURFACE('',#8437,2.5);
#7479=CYLINDRICAL_SURFACE('',#8440,1.);
#7480=CYLINDRICAL_SURFACE('',#8444,2.5);
#7481=CYLINDRICAL_SURFACE('',#8451,2.5);
#7482=CYLINDRICAL_SURFACE('',#8459,2.);
#7483=CYLINDRICAL_SURFACE('',#8460,2.);
#7484=CYLINDRICAL_SURFACE('',#8461,2.);
#7638=ADVANCED_FACE('',(#476),#7443,.T.);
#7639=ADVANCED_FACE('',(#477),#284,.T.);
#7640=ADVANCED_FACE('',(#478),#285,.F.);
#7641=ADVANCED_FACE('',(#479),#7444,.F.);
#7642=ADVANCED_FACE('',(#480),#286,.F.);
#7643=ADVANCED_FACE('',(#481),#7445,.F.);
#7644=ADVANCED_FACE('',(#482),#287,.F.);
#7645=ADVANCED_FACE('',(#483),#288,.F.);
#7646=ADVANCED_FACE('',(#484),#289,.F.);
#7647=ADVANCED_FACE('',(#485),#290,.F.);
#7648=ADVANCED_FACE('',(#486),#7446,.T.);
#7649=ADVANCED_FACE('',(#487),#7447,.T.);
#7650=ADVANCED_FACE('',(#488),#7448,.T.);
#7651=ADVANCED_FACE('',(#489),#7449,.T.);
#7652=ADVANCED_FACE('',(#490),#214,.T.);
#7653=ADVANCED_FACE('',(#491),#7450,.T.);
#7654=ADVANCED_FACE('',(#492),#215,.T.);
#7655=ADVANCED_FACE('',(#493),#7451,.T.);
#7656=ADVANCED_FACE('',(#494),#196,.T.);
#7657=ADVANCED_FACE('',(#495),#7452,.T.);
#7658=ADVANCED_FACE('',(#496),#197,.T.);
#7659=ADVANCED_FACE('',(#497),#291,.T.);
#7660=ADVANCED_FACE('',(#498),#7453,.T.);
#7661=ADVANCED_FACE('',(#499),#292,.T.);
#7662=ADVANCED_FACE('',(#500),#7454,.T.);
#7663=ADVANCED_FACE('',(#501),#293,.T.);
#7664=ADVANCED_FACE('',(#502),#294,.F.);
#7665=ADVANCED_FACE('',(#503),#295,.F.);
#7666=ADVANCED_FACE('',(#504),#7455,.F.);
#7667=ADVANCED_FACE('',(#505),#296,.F.);
#7668=ADVANCED_FACE('',(#506),#7456,.F.);
#7669=ADVANCED_FACE('',(#507),#297,.T.);
#7670=ADVANCED_FACE('',(#508),#298,.F.);
#7671=ADVANCED_FACE('',(#509),#7457,.F.);
#7672=ADVANCED_FACE('',(#510),#7458,.F.);
#7673=ADVANCED_FACE('',(#511),#7459,.F.);
#7674=ADVANCED_FACE('',(#512),#7460,.F.);
#7675=ADVANCED_FACE('',(#513),#299,.F.);
#7676=ADVANCED_FACE('',(#514),#300,.F.);
#7677=ADVANCED_FACE('',(#515),#301,.F.);
#7678=ADVANCED_FACE('',(#516),#302,.F.);
#7679=ADVANCED_FACE('',(#517),#303,.F.);
#7680=ADVANCED_FACE('',(#518),#304,.T.);
#7681=ADVANCED_FACE('',(#519),#305,.F.);
#7682=ADVANCED_FACE('',(#520),#306,.F.);
#7683=ADVANCED_FACE('',(#521),#307,.F.);
#7684=ADVANCED_FACE('',(#522),#7461,.T.);
#7685=ADVANCED_FACE('',(#523),#7462,.T.);
#7686=ADVANCED_FACE('',(#524),#308,.T.);
#7687=ADVANCED_FACE('',(#525),#309,.T.);
#7688=ADVANCED_FACE('',(#526),#310,.F.);
#7689=ADVANCED_FACE('',(#527),#311,.F.);
#7690=ADVANCED_FACE('',(#528),#7463,.T.);
#7691=ADVANCED_FACE('',(#529),#312,.T.);
#7692=ADVANCED_FACE('',(#530),#313,.T.);
#7693=ADVANCED_FACE('',(#531),#7464,.T.);
#7694=ADVANCED_FACE('',(#532),#314,.F.);
#7695=ADVANCED_FACE('',(#533),#315,.T.);
#7696=ADVANCED_FACE('',(#534),#7465,.T.);
#7697=ADVANCED_FACE('',(#535),#216,.T.);
#7698=ADVANCED_FACE('',(#536),#7466,.T.);
#7699=ADVANCED_FACE('',(#537),#217,.T.);
#7700=ADVANCED_FACE('',(#538),#7467,.T.);
#7701=ADVANCED_FACE('',(#539),#178,.F.);
#7702=ADVANCED_FACE('',(#540),#7468,.T.);
#7703=ADVANCED_FACE('',(#541),#179,.F.);
#7704=ADVANCED_FACE('',(#542),#7469,.T.);
#7705=ADVANCED_FACE('',(#543),#7470,.T.);
#7706=ADVANCED_FACE('',(#544),#218,.T.);
#7707=ADVANCED_FACE('',(#545),#198,.T.);
#7708=ADVANCED_FACE('',(#546),#199,.T.);
#7709=ADVANCED_FACE('',(#547),#200,.T.);
#7710=ADVANCED_FACE('',(#548),#201,.T.);
#7711=ADVANCED_FACE('',(#549),#7471,.T.);
#7712=ADVANCED_FACE('',(#550),#316,.F.);
#7713=ADVANCED_FACE('',(#551),#7472,.F.);
#7714=ADVANCED_FACE('',(#552),#317,.F.);
#7715=ADVANCED_FACE('',(#553),#7473,.T.);
#7716=ADVANCED_FACE('',(#554),#7474,.T.);
#7717=ADVANCED_FACE('',(#555),#7475,.T.);
#7718=ADVANCED_FACE('',(#556),#318,.T.);
#7719=ADVANCED_FACE('',(#557),#7476,.F.);
#7720=ADVANCED_FACE('',(#558),#7477,.T.);
#7721=ADVANCED_FACE('',(#559),#7478,.F.);
#7722=ADVANCED_FACE('',(#560),#319,.F.);
#7723=ADVANCED_FACE('',(#561),#7479,.T.);
#7724=ADVANCED_FACE('',(#562),#320,.F.);
#7725=ADVANCED_FACE('',(#563),#321,.F.);
#7726=ADVANCED_FACE('',(#564),#7480,.F.);
#7727=ADVANCED_FACE('',(#565,#138),#322,.T.);
#7728=ADVANCED_FACE('',(#566,#139),#323,.T.);
#7729=ADVANCED_FACE('',(#567),#324,.F.);
#7730=ADVANCED_FACE('',(#568),#7481,.F.);
#7731=ADVANCED_FACE('',(#569),#325,.F.);
#7732=ADVANCED_FACE('',(#570,#140),#326,.T.);
#7733=ADVANCED_FACE('',(#571,#141),#327,.T.);
#7734=ADVANCED_FACE('',(#572),#328,.T.);
#7735=ADVANCED_FACE('',(#573),#329,.T.);
#7736=ADVANCED_FACE('',(#574),#7482,.T.);
#7737=ADVANCED_FACE('',(#575),#7483,.T.);
#7738=ADVANCED_FACE('',(#576),#7484,.T.);
#8115=CLOSED_SHELL('',(#7638,#7639,#7640,#7641,#7642,#7643,#7644,#7645,
#7646,#7647,#7648,#7649,#7650,#7651,#7652,#7653,#7654,#7655,#7656,#7657,
#7658,#7659,#7660,#7661,#7662,#7663,#7664,#7665,#7666,#7667,#7668,#7669,
#7670,#7671,#7672,#7673,#7674,#7675,#7676,#7677,#7678,#7679,#7680,#7681,
#7682,#7683,#7684,#7685,#7686,#7687,#7688,#7689,#7690,#7691,#7692,#7693,
#7694,#7695,#7696,#7697,#7698,#7699,#7700,#7701,#7702,#7703,#7704,#7705,
#7706,#7707,#7708,#7709,#7710,#7711,#7712,#7713,#7714,#7715,#7716,#7717,
#7718,#7719,#7720,#7721,#7722,#7723,#7724,#7725,#7726,#7727,#7728,#7729,
#7730,#7731,#7732,#7733,#7734,#7735,#7736,#7737,#7738));
#8261=AXIS2_PLACEMENT_3D('',#11812,#9253,#9254);
#8262=AXIS2_PLACEMENT_3D('',#11813,#9255,#9256);
#8263=AXIS2_PLACEMENT_3D('',#11831,#9258,#9259);
#8264=AXIS2_PLACEMENT_3D('',#11835,#9261,#9262);
#8265=AXIS2_PLACEMENT_3D('',#11838,#9264,#9265);
#8266=AXIS2_PLACEMENT_3D('',#11839,#9266,#9267);
#8267=AXIS2_PLACEMENT_3D('',#11845,#9271,#9272);
#8268=AXIS2_PLACEMENT_3D('',#11855,#9278,#9279);
#8269=AXIS2_PLACEMENT_3D('',#11857,#9280,#9281);
#8270=AXIS2_PLACEMENT_3D('',#11859,#9283,#9284);
#8271=AXIS2_PLACEMENT_3D('',#11865,#9288,#9289);
#8272=AXIS2_PLACEMENT_3D('',#11867,#9290,#9291);
#8273=AXIS2_PLACEMENT_3D('',#11870,#9293,#9294);
#8274=AXIS2_PLACEMENT_3D('',#11871,#9295,#9296);
#8275=AXIS2_PLACEMENT_3D('',#11877,#9300,#9301);
#8276=AXIS2_PLACEMENT_3D('',#11883,#9305,#9306);
#8277=AXIS2_PLACEMENT_3D('',#11893,#9312,#9313);
#8278=AXIS2_PLACEMENT_3D('',#11897,#9315,#9316);
#8279=AXIS2_PLACEMENT_3D('',#11901,#9318,#9319);
#8280=AXIS2_PLACEMENT_3D('',#11911,#9324,#9325);
#8281=AXIS2_PLACEMENT_3D('',#11913,#9326,#9327);
#8282=AXIS2_PLACEMENT_3D('',#11917,#9329,#9330);
#8283=AXIS2_PLACEMENT_3D('',#11918,#9331,#9332);
#8284=AXIS2_PLACEMENT_3D('',#11919,#9333,#9334);
#8285=AXIS2_PLACEMENT_3D('',#11922,#9335,#9336);
#8286=AXIS2_PLACEMENT_3D('',#11926,#9338,#9339);
#8287=AXIS2_PLACEMENT_3D('',#11928,#9341,#9342);
#8288=AXIS2_PLACEMENT_3D('',#11933,#9344,#9345);
#8289=AXIS2_PLACEMENT_3D('',#11936,#9347,#9348);
#8290=AXIS2_PLACEMENT_3D('',#11937,#9349,#9350);
#8291=AXIS2_PLACEMENT_3D('',#11941,#9352,#9353);
#8292=AXIS2_PLACEMENT_3D('',#11943,#9355,#9356);
#8293=AXIS2_PLACEMENT_3D('',#11945,#9357,#9358);
#8294=AXIS2_PLACEMENT_3D('',#11949,#9360,#9361);
#8295=AXIS2_PLACEMENT_3D('',#11951,#9363,#9364);
#8296=AXIS2_PLACEMENT_3D('',#11954,#9365,#9366);
#8297=AXIS2_PLACEMENT_3D('',#11955,#9367,#9368);
#8298=AXIS2_PLACEMENT_3D('',#11956,#9369,#9370);
#8299=AXIS2_PLACEMENT_3D('',#11957,#9371,#9372);
#8300=AXIS2_PLACEMENT_3D('',#11960,#9375,#9376);
#8301=AXIS2_PLACEMENT_3D('',#11963,#9377,#9378);
#8302=AXIS2_PLACEMENT_3D('',#11964,#9379,#9380);
#8303=AXIS2_PLACEMENT_3D('',#11965,#9381,#9382);
#8304=AXIS2_PLACEMENT_3D('',#11966,#9383,#9384);
#8305=AXIS2_PLACEMENT_3D('',#11969,#9385,#9386);
#8306=AXIS2_PLACEMENT_3D('',#11972,#9389,#9390);
#8307=AXIS2_PLACEMENT_3D('',#11973,#9391,#9392);
#8308=AXIS2_PLACEMENT_3D('',#11974,#9393,#9394);
#8309=AXIS2_PLACEMENT_3D('',#11976,#9395,#9396);
#8310=AXIS2_PLACEMENT_3D('',#11980,#9398,#9399);
#8311=AXIS2_PLACEMENT_3D('',#11982,#9401,#9402);
#8312=AXIS2_PLACEMENT_3D('',#11983,#9403,#9404);
#8313=AXIS2_PLACEMENT_3D('',#11984,#9405,#9406);
#8314=AXIS2_PLACEMENT_3D('',#11999,#9415,#9416);
#8315=AXIS2_PLACEMENT_3D('',#12002,#9418,#9419);
#8316=AXIS2_PLACEMENT_3D('',#12003,#9420,#9421);
#8317=AXIS2_PLACEMENT_3D('',#12009,#9424,#9425);
#8318=AXIS2_PLACEMENT_3D('',#12011,#9426,#9427);
#8319=AXIS2_PLACEMENT_3D('',#12015,#9429,#9430);
#8320=AXIS2_PLACEMENT_3D('',#12019,#9432,#9433);
#8321=AXIS2_PLACEMENT_3D('',#12025,#9436,#9437);
#8322=AXIS2_PLACEMENT_3D('',#12027,#9439,#9440);
#8323=AXIS2_PLACEMENT_3D('',#12030,#9442,#9443);
#8324=AXIS2_PLACEMENT_3D('',#12031,#9444,#9445);
#8325=AXIS2_PLACEMENT_3D('',#12043,#9452,#9453);
#8326=AXIS2_PLACEMENT_3D('',#12052,#9458,#9459);
#8327=AXIS2_PLACEMENT_3D('',#12061,#9464,#9465);
#8328=AXIS2_PLACEMENT_3D('',#12062,#9466,#9467);
#8329=AXIS2_PLACEMENT_3D('',#12063,#9468,#9469);
#8330=AXIS2_PLACEMENT_3D('',#12064,#9470,#9471);
#8331=AXIS2_PLACEMENT_3D('',#12070,#9475,#9476);
#8332=AXIS2_PLACEMENT_3D('',#12071,#9477,#9478);
#8333=AXIS2_PLACEMENT_3D('',#12072,#9479,#9480);
#8334=AXIS2_PLACEMENT_3D('',#12073,#9481,#9482);
#8335=AXIS2_PLACEMENT_3D('',#12081,#9487,#9488);
#8336=AXIS2_PLACEMENT_3D('',#12083,#9489,#9490);
#8337=AXIS2_PLACEMENT_3D('',#12087,#9492,#9493);
#8338=AXIS2_PLACEMENT_3D('',#12091,#9495,#9496);
#8339=AXIS2_PLACEMENT_3D('',#12096,#9499,#9500);
#8340=AXIS2_PLACEMENT_3D('',#12100,#9502,#9503);
#8341=AXIS2_PLACEMENT_3D('',#12103,#9505,#9506);
#8342=AXIS2_PLACEMENT_3D('',#12105,#9507,#9508);
#8343=AXIS2_PLACEMENT_3D('',#12107,#9510,#9511);
#8344=AXIS2_PLACEMENT_3D('',#12109,#9512,#9513);
#8345=AXIS2_PLACEMENT_3D('',#12113,#9515,#9516);
#8346=AXIS2_PLACEMENT_3D('',#12117,#9519,#9520);
#8347=AXIS2_PLACEMENT_3D('',#12118,#9521,#9522);
#8348=AXIS2_PLACEMENT_3D('',#12120,#9523,#9524);
#8349=AXIS2_PLACEMENT_3D('',#12124,#9526,#9527);
#8350=AXIS2_PLACEMENT_3D('',#12126,#9529,#9530);
#8351=AXIS2_PLACEMENT_3D('',#12127,#9531,#9532);
#8352=AXIS2_PLACEMENT_3D('',#12129,#9533,#9534);
#8353=AXIS2_PLACEMENT_3D('',#12134,#9537,#9538);
#8354=AXIS2_PLACEMENT_3D('',#12136,#9540,#9541);
#8355=AXIS2_PLACEMENT_3D('',#12138,#9542,#9543);
#8356=AXIS2_PLACEMENT_3D('',#12142,#9546,#9547);
#8357=AXIS2_PLACEMENT_3D('',#12143,#9548,#9549);
#8358=AXIS2_PLACEMENT_3D('',#12147,#9552,#9553);
#8359=AXIS2_PLACEMENT_3D('',#12151,#9556,#9557);
#8360=AXIS2_PLACEMENT_3D('',#12157,#9560,#9561);
#8361=AXIS2_PLACEMENT_3D('',#12161,#9564,#9565);
#8362=AXIS2_PLACEMENT_3D('',#12167,#9569,#9570);
#8363=AXIS2_PLACEMENT_3D('',#12175,#9575,#9576);
#8364=AXIS2_PLACEMENT_3D('',#12179,#9579,#9580);
#8365=AXIS2_PLACEMENT_3D('',#12183,#9583,#9584);
#8366=AXIS2_PLACEMENT_3D('',#12186,#9585,#9586);
#8367=AXIS2_PLACEMENT_3D('',#12195,#9591,#9592);
#8368=AXIS2_PLACEMENT_3D('',#12199,#9595,#9596);
#8369=AXIS2_PLACEMENT_3D('',#12202,#9598,#9599);
#8370=AXIS2_PLACEMENT_3D('',#12203,#9600,#9601);
#8371=AXIS2_PLACEMENT_3D('',#12205,#9603,#9604);
#8372=AXIS2_PLACEMENT_3D('',#12207,#9605,#9606);
#8373=AXIS2_PLACEMENT_3D('',#12209,#9608,#9609);
#8374=AXIS2_PLACEMENT_3D('',#12211,#9610,#9611);
#8375=AXIS2_PLACEMENT_3D('',#12213,#9613,#9614);
#8376=AXIS2_PLACEMENT_3D('',#12215,#9616,#9617);
#8377=AXIS2_PLACEMENT_3D('',#12219,#9620,#9621);
#8378=AXIS2_PLACEMENT_3D('',#12221,#9623,#9624);
#8379=AXIS2_PLACEMENT_3D('',#12223,#9626,#9627);
#8380=AXIS2_PLACEMENT_3D('',#12224,#9628,#9629);
#8381=AXIS2_PLACEMENT_3D('',#12228,#9632,#9633);
#8382=AXIS2_PLACEMENT_3D('',#12232,#9636,#9637);
#8383=AXIS2_PLACEMENT_3D('',#12233,#9638,#9639);
#8384=AXIS2_PLACEMENT_3D('',#12234,#9640,#9641);
#8385=AXIS2_PLACEMENT_3D('',#12235,#9642,#9643);
#8386=AXIS2_PLACEMENT_3D('',#12236,#9644,#9645);
#8387=AXIS2_PLACEMENT_3D('',#12238,#9646,#9647);
#8388=AXIS2_PLACEMENT_3D('',#12241,#9649,#9650);
#8389=AXIS2_PLACEMENT_3D('',#12242,#9651,#9652);
#8390=AXIS2_PLACEMENT_3D('',#12244,#9653,#9654);
#8391=AXIS2_PLACEMENT_3D('',#12245,#9655,#9656);
#8392=AXIS2_PLACEMENT_3D('',#12246,#9657,#9658);
#8393=AXIS2_PLACEMENT_3D('',#12248,#9659,#9660);
#8394=AXIS2_PLACEMENT_3D('',#12250,#9662,#9663);
#8395=AXIS2_PLACEMENT_3D('',#12252,#9664,#9665);
#8396=AXIS2_PLACEMENT_3D('',#12254,#9666,#9667);
#8397=AXIS2_PLACEMENT_3D('',#12255,#9668,#9669);
#8398=AXIS2_PLACEMENT_3D('',#12256,#9670,#9671);
#8399=AXIS2_PLACEMENT_3D('',#12258,#9672,#9673);
#8400=AXIS2_PLACEMENT_3D('',#12269,#9675,#9676);
#8401=AXIS2_PLACEMENT_3D('',#12270,#9677,#9678);
#8402=AXIS2_PLACEMENT_3D('',#12271,#9679,#9680);
#8403=AXIS2_PLACEMENT_3D('',#12272,#9681,#9682);
#8404=AXIS2_PLACEMENT_3D('',#12282,#9683,#9684);
#8405=AXIS2_PLACEMENT_3D('',#12283,#9685,#9686);
#8406=AXIS2_PLACEMENT_3D('',#12284,#9687,#9688);
#8407=AXIS2_PLACEMENT_3D('',#12285,#9689,#9690);
#8408=AXIS2_PLACEMENT_3D('',#12286,#9691,#9692);
#8409=AXIS2_PLACEMENT_3D('',#12288,#9693,#9694);
#8410=AXIS2_PLACEMENT_3D('',#12291,#9696,#9697);
#8411=AXIS2_PLACEMENT_3D('',#12292,#9698,#9699);
#8412=AXIS2_PLACEMENT_3D('',#12294,#9700,#9701);
#8413=AXIS2_PLACEMENT_3D('',#12295,#9702,#9703);
#8414=AXIS2_PLACEMENT_3D('',#12296,#9704,#9705);
#8415=AXIS2_PLACEMENT_3D('',#12297,#9706,#9707);
#8416=AXIS2_PLACEMENT_3D('',#12298,#9708,#9709);
#8417=AXIS2_PLACEMENT_3D('',#12299,#9710,#9711);
#8418=AXIS2_PLACEMENT_3D('',#12300,#9712,#9713);
#8419=AXIS2_PLACEMENT_3D('',#12301,#9714,#9715);
#8420=AXIS2_PLACEMENT_3D('',#12302,#9716,#9717);
#8421=AXIS2_PLACEMENT_3D('',#12303,#9718,#9719);
#8422=AXIS2_PLACEMENT_3D('',#12304,#9720,#9721);
#8423=AXIS2_PLACEMENT_3D('',#12307,#9723,#9724);
#8424=AXIS2_PLACEMENT_3D('',#12308,#9725,#9726);
#8425=AXIS2_PLACEMENT_3D('',#12312,#9729,#9730);
#8426=AXIS2_PLACEMENT_3D('',#12315,#9732,#9733);
#8427=AXIS2_PLACEMENT_3D('',#12316,#9734,#9735);
#8428=AXIS2_PLACEMENT_3D('',#12320,#9738,#9739);
#8429=AXIS2_PLACEMENT_3D('',#12321,#9740,#9741);
#8430=AXIS2_PLACEMENT_3D('',#12322,#9742,#9743);
#8431=AXIS2_PLACEMENT_3D('',#12323,#9744,#9745);
#8432=AXIS2_PLACEMENT_3D('',#12325,#9747,#9748);
#8433=AXIS2_PLACEMENT_3D('',#12327,#9750,#9751);
#8434=AXIS2_PLACEMENT_3D('',#12331,#9753,#9754);
#8435=AXIS2_PLACEMENT_3D('',#12333,#9756,#9757);
#8436=AXIS2_PLACEMENT_3D('',#12336,#9759,#9760);
#8437=AXIS2_PLACEMENT_3D('',#12337,#9761,#9762);
#8438=AXIS2_PLACEMENT_3D('',#12340,#9764,#9765);
#8439=AXIS2_PLACEMENT_3D('',#12341,#9766,#9767);
#8440=AXIS2_PLACEMENT_3D('',#12345,#9770,#9771);
#8441=AXIS2_PLACEMENT_3D('',#12346,#9772,#9773);
#8442=AXIS2_PLACEMENT_3D('',#12347,#9774,#9775);
#8443=AXIS2_PLACEMENT_3D('',#12351,#9778,#9779);
#8444=AXIS2_PLACEMENT_3D('',#12357,#9783,#9784);
#8445=AXIS2_PLACEMENT_3D('',#12358,#9785,#9786);
#8446=AXIS2_PLACEMENT_3D('',#12359,#9787,#9788);
#8447=AXIS2_PLACEMENT_3D('',#12361,#9789,#9790);
#8448=AXIS2_PLACEMENT_3D('',#12363,#9792,#9793);
#8449=AXIS2_PLACEMENT_3D('',#12366,#9795,#9796);
#8450=AXIS2_PLACEMENT_3D('',#12367,#9797,#9798);
#8451=AXIS2_PLACEMENT_3D('',#12371,#9801,#9802);
#8452=AXIS2_PLACEMENT_3D('',#12374,#9804,#9805);
#8453=AXIS2_PLACEMENT_3D('',#12375,#9806,#9807);
#8454=AXIS2_PLACEMENT_3D('',#12379,#9810,#9811);
#8455=AXIS2_PLACEMENT_3D('',#12382,#9813,#9814);
#8456=AXIS2_PLACEMENT_3D('',#12383,#9815,#9816);
#8457=AXIS2_PLACEMENT_3D('',#12384,#9817,#9818);
#8458=AXIS2_PLACEMENT_3D('',#12386,#9820,#9821);
#8459=AXIS2_PLACEMENT_3D('',#12389,#9824,#9825);
#8460=AXIS2_PLACEMENT_3D('',#12390,#9826,#9827);
#8461=AXIS2_PLACEMENT_3D('',#12391,#9828,#9829);
#9253=DIRECTION('axis',(0.,0.,1.));
#9254=DIRECTION('refdir',(1.,0.,0.));
#9255=DIRECTION('center_axis',(-1.,0.,0.));
#9256=DIRECTION('ref_axis',(0.,0.,1.));
#9257=DIRECTION('',(1.,0.,0.));
#9258=DIRECTION('center_axis',(1.,-9.61038138866416E-16,0.));
#9259=DIRECTION('ref_axis',(0.,0.,1.));
#9260=DIRECTION('',(-1.,0.,0.));
#9261=DIRECTION('center_axis',(1.,0.,0.));
#9262=DIRECTION('ref_axis',(0.,0.,1.));
#9263=DIRECTION('',(-1.,0.,0.));
#9264=DIRECTION('center_axis',(-1.,0.,0.));
#9265=DIRECTION('ref_axis',(0.,0.,1.));
#9266=DIRECTION('center_axis',(0.,-1.,0.));
#9267=DIRECTION('ref_axis',(0.,0.,1.));
#9268=DIRECTION('',(0.,0.,-1.));
#9269=DIRECTION('',(1.,0.,0.));
#9270=DIRECTION('',(0.,0.,-1.));
#9271=DIRECTION('center_axis',(0.,1.,0.));
#9272=DIRECTION('ref_axis',(-1.,0.,0.));
#9273=DIRECTION('',(0.,0.,1.));
#9274=DIRECTION('',(-1.,0.,0.));
#9275=DIRECTION('',(0.,0.,1.));
#9276=DIRECTION('',(0.,0.,1.));
#9277=DIRECTION('',(1.,0.,0.));
#9278=DIRECTION('center_axis',(0.,0.,1.));
#9279=DIRECTION('ref_axis',(-2.22044604925031E-15,1.,0.));
#9280=DIRECTION('center_axis',(0.,0.,1.));
#9281=DIRECTION('ref_axis',(-2.22044604925031E-15,1.,0.));
#9282=DIRECTION('',(0.,0.,1.));
#9283=DIRECTION('center_axis',(1.,0.,0.));
#9284=DIRECTION('ref_axis',(0.,1.,0.));
#9285=DIRECTION('',(0.,1.,0.));
#9286=DIRECTION('',(0.,0.,1.));
#9287=DIRECTION('',(0.,-1.,0.));
#9288=DIRECTION('center_axis',(0.,0.,1.));
#9289=DIRECTION('ref_axis',(1.,2.22044604925032E-15,0.));
#9290=DIRECTION('center_axis',(0.,0.,1.));
#9291=DIRECTION('ref_axis',(1.,2.22044604925032E-15,0.));
#9292=DIRECTION('',(0.,0.,1.));
#9293=DIRECTION('center_axis',(0.,0.,-1.));
#9294=DIRECTION('ref_axis',(1.,2.22044604925032E-15,0.));
#9295=DIRECTION('center_axis',(0.,-1.,0.));
#9296=DIRECTION('ref_axis',(1.,0.,0.));
#9297=DIRECTION('',(0.,0.,-1.));
#9298=DIRECTION('',(-1.,0.,0.));
#9299=DIRECTION('',(1.,0.,0.));
#9300=DIRECTION('center_axis',(0.,0.,-1.));
#9301=DIRECTION('ref_axis',(0.,1.,0.));
#9302=DIRECTION('',(0.,1.,0.));
#9303=DIRECTION('',(-1.,0.,0.));
#9304=DIRECTION('',(0.,1.,0.));
#9305=DIRECTION('center_axis',(0.,0.,-1.));
#9306=DIRECTION('ref_axis',(0.,1.,0.));
#9307=DIRECTION('',(0.,1.,0.));
#9308=DIRECTION('',(1.,0.,0.));
#9309=DIRECTION('',(0.,1.,0.));
#9310=DIRECTION('',(-1.,0.,0.));
#9311=DIRECTION('',(0.,1.,0.));
#9312=DIRECTION('center_axis',(1.,0.,0.));
#9313=DIRECTION('ref_axis',(0.,1.,0.));
#9314=DIRECTION('',(0.,1.,0.));
#9315=DIRECTION('center_axis',(1.,0.,0.));
#9316=DIRECTION('ref_axis',(0.,-1.,0.));
#9317=DIRECTION('',(0.,0.,-1.));
#9318=DIRECTION('center_axis',(1.,0.,0.));
#9319=DIRECTION('ref_axis',(0.,-0.707106781186549,0.707106781186546));
#9320=DIRECTION('',(0.,-1.,0.));
#9321=DIRECTION('',(0.,0.,-1.));
#9322=DIRECTION('',(0.,-1.,0.));
#9323=DIRECTION('',(0.,0.,-1.));
#9324=DIRECTION('center_axis',(1.,0.,0.));
#9325=DIRECTION('ref_axis',(0.,1.,0.));
#9326=DIRECTION('center_axis',(1.,0.,0.));
#9327=DIRECTION('ref_axis',(0.,1.,0.));
#9328=DIRECTION('',(0.,0.,-1.));
#9329=DIRECTION('center_axis',(1.,0.,0.));
#9330=DIRECTION('ref_axis',(0.,1.,0.));
#9331=DIRECTION('center_axis',(1.,0.,0.));
#9332=DIRECTION('ref_axis',(0.,1.,0.));
#9333=DIRECTION('center_axis',(1.,0.,0.));
#9334=DIRECTION('ref_axis',(0.,-0.707106781186548,-0.707106781186547));
#9335=DIRECTION('center_axis',(-1.,0.,0.));
#9336=DIRECTION('ref_axis',(0.,0.,-1.));
#9337=DIRECTION('',(-1.,0.,0.));
#9338=DIRECTION('center_axis',(-1.,0.,0.));
#9339=DIRECTION('ref_axis',(0.,-0.707106781186548,-0.707106781186547));
#9340=DIRECTION('',(1.,0.,0.));
#9341=DIRECTION('center_axis',(0.,0.,1.));
#9342=DIRECTION('ref_axis',(0.707106781186548,0.707106781186548,0.));
#9343=DIRECTION('',(0.,0.,1.));
#9344=DIRECTION('center_axis',(0.,-5.55111512312576E-16,-1.));
#9345=DIRECTION('ref_axis',(0.,1.,-5.55111512312577E-16));
#9346=DIRECTION('',(0.,0.,-1.));
#9347=DIRECTION('center_axis',(0.,0.707106781186548,0.707106781186548));
#9348=DIRECTION('ref_axis',(0.,0.707106781186548,-0.707106781186548));
#9349=DIRECTION('center_axis',(0.,1.,0.));
#9350=DIRECTION('ref_axis',(0.707106781186548,0.,-0.707106781186548));
#9351=DIRECTION('',(0.,-1.,0.));
#9352=DIRECTION('center_axis',(0.,0.707106781186548,-0.707106781186547));
#9353=DIRECTION('ref_axis',(0.,-0.707106781186547,-0.707106781186548));
#9354=DIRECTION('',(0.,1.,0.));
#9355=DIRECTION('center_axis',(0.,1.,0.));
#9356=DIRECTION('ref_axis',(0.707106781186548,0.,-0.707106781186547));
#9357=DIRECTION('center_axis',(0.,1.,0.));
#9358=DIRECTION('ref_axis',(1.,0.,0.));
#9359=DIRECTION('',(0.,1.,0.));
#9360=DIRECTION('center_axis',(0.,-1.,0.));
#9361=DIRECTION('ref_axis',(0.,0.,-1.));
#9362=DIRECTION('',(0.,-1.,0.));
#9363=DIRECTION('center_axis',(-1.,0.,0.));
#9364=DIRECTION('ref_axis',(0.,0.,1.));
#9365=DIRECTION('center_axis',(0.,-5.55111512312578E-16,1.));
#9366=DIRECTION('ref_axis',(0.,-1.,-5.55111512312578E-16));
#9367=DIRECTION('center_axis',(1.,0.,0.));
#9368=DIRECTION('ref_axis',(0.,0.707106781186548,0.707106781186548));
#9369=DIRECTION('center_axis',(-1.,0.,0.));
#9370=DIRECTION('ref_axis',(0.,0.707106781186548,0.707106781186548));
#9371=DIRECTION('center_axis',(0.,0.,-1.));
#9372=DIRECTION('ref_axis',(0.707106781186548,-0.707106781186548,0.));
#9373=DIRECTION('',(0.,0.,1.));
#9374=DIRECTION('',(0.,0.,-1.));
#9375=DIRECTION('center_axis',(-1.,0.,0.));
#9376=DIRECTION('ref_axis',(0.,0.,1.));
#9377=DIRECTION('center_axis',(0.,-1.,0.));
#9378=DIRECTION('ref_axis',(0.,0.,-1.));
#9379=DIRECTION('center_axis',(1.,0.,0.));
#9380=DIRECTION('ref_axis',(0.,-0.707106781186548,0.707106781186547));
#9381=DIRECTION('center_axis',(-1.,0.,0.));
#9382=DIRECTION('ref_axis',(0.,-0.707106781186548,0.707106781186547));
#9383=DIRECTION('center_axis',(0.,1.,0.));
#9384=DIRECTION('ref_axis',(0.707106781186548,0.,-0.707106781186547));
#9385=DIRECTION('center_axis',(0.,-1.,0.));
#9386=DIRECTION('ref_axis',(0.,0.,-1.));
#9387=DIRECTION('',(0.,-1.,0.));
#9388=DIRECTION('',(0.,1.,0.));
#9389=DIRECTION('center_axis',(-0.816496580927725,-0.408248290463864,-0.408248290463863));
#9390=DIRECTION('ref_axis',(0.577350269189626,-0.577350269189626,-0.577350269189625));
#9391=DIRECTION('center_axis',(0.,0.,-1.));
#9392=DIRECTION('ref_axis',(0.707106781186548,-0.707106781186548,0.));
#9393=DIRECTION('center_axis',(-1.,0.,0.));
#9394=DIRECTION('ref_axis',(0.,0.707106781186547,-0.707106781186548));
#9395=DIRECTION('center_axis',(-1.,0.,0.));
#9396=DIRECTION('ref_axis',(0.,1.,1.11022302462516E-15));
#9397=DIRECTION('',(-1.,0.,0.));
#9398=DIRECTION('center_axis',(-1.,0.,0.));
#9399=DIRECTION('ref_axis',(0.,0.707106781186547,-0.707106781186548));
#9400=DIRECTION('',(1.,0.,0.));
#9401=DIRECTION('center_axis',(-0.816496580927726,0.408248290463863,-0.408248290463863));
#9402=DIRECTION('ref_axis',(0.577350269189628,0.577350269189627,-0.577350269189623));
#9403=DIRECTION('center_axis',(0.,0.,-1.));
#9404=DIRECTION('ref_axis',(0.707106781186549,0.707106781186546,0.));
#9405=DIRECTION('center_axis',(0.,-1.,0.));
#9406=DIRECTION('ref_axis',(0.,0.,-1.));
#9407=DIRECTION('',(0.,0.,1.));
#9408=DIRECTION('',(0.,0.,-1.));
#9409=DIRECTION('',(1.,0.,0.));
#9410=DIRECTION('',(0.,0.,1.));
#9411=DIRECTION('',(-1.,0.,0.));
#9412=DIRECTION('',(0.,0.,-1.));
#9413=DIRECTION('',(1.,0.,0.));
#9414=DIRECTION('',(1.,0.,0.));
#9415=DIRECTION('center_axis',(0.,0.,-1.));
#9416=DIRECTION('ref_axis',(0.707106781186548,-0.707106781186548,0.));
#9417=DIRECTION('',(0.,0.,1.));
#9418=DIRECTION('center_axis',(0.,0.,-1.));
#9419=DIRECTION('ref_axis',(1.,0.,0.));
#9420=DIRECTION('center_axis',(1.,0.,0.));
#9421=DIRECTION('ref_axis',(0.,1.,0.));
#9422=DIRECTION('',(0.,0.,-1.));
#9423=DIRECTION('',(0.,1.,0.));
#9424=DIRECTION('center_axis',(1.,0.,0.));
#9425=DIRECTION('ref_axis',(0.,-0.847202876515606,-0.531269504134844));
#9426=DIRECTION('center_axis',(1.,0.,0.));
#9427=DIRECTION('ref_axis',(0.,-0.790280212002226,-0.612745613217848));
#9428=DIRECTION('',(0.,-2.79713066068216E-16,-1.));
#9429=DIRECTION('center_axis',(-1.,0.,0.));
#9430=DIRECTION('ref_axis',(0.,0.707106781186548,0.707106781186547));
#9431=DIRECTION('',(0.,1.,0.));
#9432=DIRECTION('center_axis',(-1.,0.,0.));
#9433=DIRECTION('ref_axis',(0.,-0.707106781186549,0.707106781186546));
#9434=DIRECTION('',(0.,0.,1.));
#9435=DIRECTION('',(0.,-1.,0.));
#9436=DIRECTION('center_axis',(1.,0.,0.));
#9437=DIRECTION('ref_axis',(0.,1.,0.));
#9438=DIRECTION('',(0.,1.,0.));
#9439=DIRECTION('center_axis',(0.,0.,1.));
#9440=DIRECTION('ref_axis',(0.707106781186549,0.707106781186546,0.));
#9441=DIRECTION('',(0.,0.,1.));
#9442=DIRECTION('center_axis',(0.,0.,-1.));
#9443=DIRECTION('ref_axis',(0.,1.,0.));
#9444=DIRECTION('center_axis',(0.,1.,0.));
#9445=DIRECTION('ref_axis',(0.,0.,1.));
#9446=DIRECTION('',(0.,0.,-1.));
#9447=DIRECTION('',(1.,0.,0.));
#9448=DIRECTION('',(0.,0.,1.));
#9449=DIRECTION('',(1.,0.,0.));
#9450=DIRECTION('',(0.,0.,-1.));
#9451=DIRECTION('',(-1.,0.,0.));
#9452=DIRECTION('center_axis',(0.,1.,0.));
#9453=DIRECTION('ref_axis',(1.,0.,0.));
#9454=DIRECTION('',(-1.,0.,0.));
#9455=DIRECTION('',(0.,0.,-1.));
#9456=DIRECTION('',(1.,0.,0.));
#9457=DIRECTION('',(0.,0.,1.));
#9458=DIRECTION('center_axis',(1.,0.,0.));
#9459=DIRECTION('ref_axis',(0.,-1.,0.));
#9460=DIRECTION('',(0.,1.,0.));
#9461=DIRECTION('',(0.,0.,-1.));
#9462=DIRECTION('',(0.,-1.,0.));
#9463=DIRECTION('',(0.,0.,-1.));
#9464=DIRECTION('center_axis',(0.,0.,-1.));
#9465=DIRECTION('ref_axis',(1.,-1.11022302462516E-15,0.));
#9466=DIRECTION('center_axis',(0.,0.,1.));
#9467=DIRECTION('ref_axis',(1.,-1.11022302462516E-15,0.));
#9468=DIRECTION('center_axis',(0.,0.,-1.));
#9469=DIRECTION('ref_axis',(1.,-1.11022302462516E-15,0.));
#9470=DIRECTION('center_axis',(-1.11022302462516E-16,-1.,0.));
#9471=DIRECTION('ref_axis',(-1.,1.11022302462516E-16,0.));
#9472=DIRECTION('',(1.,-1.11022302462516E-16,0.));
#9473=DIRECTION('',(-1.,1.11022302462516E-16,0.));
#9474=DIRECTION('',(0.,0.,-1.));
#9475=DIRECTION('center_axis',(0.,0.,-1.));
#9476=DIRECTION('ref_axis',(0.,-1.,0.));
#9477=DIRECTION('center_axis',(0.,0.,1.));
#9478=DIRECTION('ref_axis',(0.,-1.,0.));
#9479=DIRECTION('center_axis',(0.,0.,-1.));
#9480=DIRECTION('ref_axis',(0.,-1.,0.));
#9481=DIRECTION('center_axis',(0.,0.,1.));
#9482=DIRECTION('ref_axis',(0.,-1.,0.));
#9483=DIRECTION('',(-1.,0.,0.));
#9484=DIRECTION('',(0.,-1.,0.));
#9485=DIRECTION('',(1.,0.,0.));
#9486=DIRECTION('',(0.,-1.,0.));
#9487=DIRECTION('center_axis',(1.,0.,0.));
#9488=DIRECTION('ref_axis',(0.,1.,0.));
#9489=DIRECTION('center_axis',(1.,0.,0.));
#9490=DIRECTION('ref_axis',(0.,1.,0.));
#9491=DIRECTION('',(0.,0.,1.));
#9492=DIRECTION('center_axis',(1.,0.,0.));
#9493=DIRECTION('ref_axis',(0.,1.,0.));
#9494=DIRECTION('',(0.,-1.,0.));
#9495=DIRECTION('center_axis',(-1.,0.,0.));
#9496=DIRECTION('ref_axis',(0.,-1.,0.));
#9497=DIRECTION('',(0.,2.79713066068216E-16,1.));
#9498=DIRECTION('',(0.,-1.,0.));
#9499=DIRECTION('center_axis',(1.,0.,0.));
#9500=DIRECTION('ref_axis',(0.,0.707106781186548,0.707106781186547));
#9501=DIRECTION('',(0.,2.79713066068216E-16,1.));
#9502=DIRECTION('center_axis',(-1.,0.,0.));
#9503=DIRECTION('ref_axis',(0.,-1.,0.));
#9504=DIRECTION('',(0.,-1.,0.));
#9505=DIRECTION('center_axis',(1.,0.,0.));
#9506=DIRECTION('ref_axis',(0.,1.,-4.44089209850062E-15));
#9507=DIRECTION('center_axis',(1.,0.,0.));
#9508=DIRECTION('ref_axis',(0.,-1.11022302462516E-15,-1.));
#9509=DIRECTION('',(0.,1.,0.));
#9510=DIRECTION('center_axis',(-1.,0.,0.));
#9511=DIRECTION('ref_axis',(0.,1.,0.));
#9512=DIRECTION('center_axis',(-1.,0.,0.));
#9513=DIRECTION('ref_axis',(0.,1.,0.));
#9514=DIRECTION('',(-1.,0.,0.));
#9515=DIRECTION('center_axis',(1.,0.,0.));
#9516=DIRECTION('ref_axis',(0.,1.,0.));
#9517=DIRECTION('',(1.,0.,0.));
#9518=DIRECTION('',(-1.,0.,0.));
#9519=DIRECTION('center_axis',(1.,0.,0.));
#9520=DIRECTION('ref_axis',(0.,1.,0.));
#9521=DIRECTION('center_axis',(-1.,0.,0.));
#9522=DIRECTION('ref_axis',(0.,1.,0.));
#9523=DIRECTION('center_axis',(-1.,0.,0.));
#9524=DIRECTION('ref_axis',(0.,1.,0.));
#9525=DIRECTION('',(-1.,0.,0.));
#9526=DIRECTION('center_axis',(1.,0.,0.));
#9527=DIRECTION('ref_axis',(0.,1.,0.));
#9528=DIRECTION('',(1.,0.,0.));
#9529=DIRECTION('center_axis',(1.,0.,0.));
#9530=DIRECTION('ref_axis',(0.,1.,0.));
#9531=DIRECTION('center_axis',(-1.,0.,0.));
#9532=DIRECTION('ref_axis',(0.,1.,0.));
#9533=DIRECTION('center_axis',(-1.,0.,0.));
#9534=DIRECTION('ref_axis',(0.,1.,0.));
#9535=DIRECTION('',(-1.,0.,0.));
#9536=DIRECTION('',(-1.,0.,0.));
#9537=DIRECTION('center_axis',(1.,0.,0.));
#9538=DIRECTION('ref_axis',(0.,1.,0.));
#9539=DIRECTION('',(1.,0.,0.));
#9540=DIRECTION('center_axis',(-1.,0.,0.));
#9541=DIRECTION('ref_axis',(0.,1.,0.));
#9542=DIRECTION('center_axis',(-1.,0.,0.));
#9543=DIRECTION('ref_axis',(0.,1.,0.));
#9544=DIRECTION('',(-1.,0.,0.));
#9545=DIRECTION('',(-1.,0.,0.));
#9546=DIRECTION('center_axis',(1.,0.,0.));
#9547=DIRECTION('ref_axis',(0.,1.,0.));
#9548=DIRECTION('center_axis',(0.,0.,1.));
#9549=DIRECTION('ref_axis',(0.,-1.,0.));
#9550=DIRECTION('',(0.,-1.,0.));
#9551=DIRECTION('',(1.,0.,0.));
#9552=DIRECTION('center_axis',(1.,0.,0.));
#9553=DIRECTION('ref_axis',(0.,1.,0.));
#9554=DIRECTION('',(0.,1.,0.));
#9555=DIRECTION('',(0.,0.,-1.));
#9556=DIRECTION('center_axis',(1.,0.,0.));
#9557=DIRECTION('ref_axis',(0.,1.,0.));
#9558=DIRECTION('',(0.,0.,1.));
#9559=DIRECTION('',(0.,1.,0.));
#9560=DIRECTION('center_axis',(-1.,0.,0.));
#9561=DIRECTION('ref_axis',(0.,0.,-1.));
#9562=DIRECTION('',(0.,-1.,0.));
#9563=DIRECTION('',(0.,0.,1.));
#9564=DIRECTION('center_axis',(0.,-1.,0.));
#9565=DIRECTION('ref_axis',(0.,0.,-1.));
#9566=DIRECTION('',(1.,0.,0.));
#9567=DIRECTION('',(0.,0.,1.));
#9568=DIRECTION('',(1.,0.,0.));
#9569=DIRECTION('center_axis',(0.,-1.,0.));
#9570=DIRECTION('ref_axis',(0.,0.,-1.));
#9571=DIRECTION('',(1.,0.,0.));
#9572=DIRECTION('',(0.,0.,1.));
#9573=DIRECTION('',(-1.,0.,0.));
#9574=DIRECTION('',(0.,0.,1.));
#9575=DIRECTION('center_axis',(0.,0.,1.));
#9576=DIRECTION('ref_axis',(0.,1.,0.));
#9577=DIRECTION('',(0.,-1.,0.));
#9578=DIRECTION('',(-1.,0.,0.));
#9579=DIRECTION('center_axis',(0.,0.,1.));
#9580=DIRECTION('ref_axis',(0.,-1.,0.));
#9581=DIRECTION('',(1.,0.,0.));
#9582=DIRECTION('',(0.,1.,0.));
#9583=DIRECTION('center_axis',(1.,0.,0.));
#9584=DIRECTION('ref_axis',(0.,1.,0.));
#9585=DIRECTION('center_axis',(1.,0.,0.));
#9586=DIRECTION('ref_axis',(0.,0.,1.));
#9587=DIRECTION('',(0.,1.,0.));
#9588=DIRECTION('',(0.,0.,-1.));
#9589=DIRECTION('',(0.,-1.,0.));
#9590=DIRECTION('',(0.,0.,1.));
#9591=DIRECTION('center_axis',(1.,0.,0.));
#9592=DIRECTION('ref_axis',(0.,1.,0.));
#9593=DIRECTION('',(0.,-1.,0.));
#9594=DIRECTION('',(0.,1.,0.));
#9595=DIRECTION('center_axis',(1.,0.,0.));
#9596=DIRECTION('ref_axis',(0.,0.,-1.));
#9597=DIRECTION('',(0.,-2.79713066068216E-16,-1.));
#9598=DIRECTION('center_axis',(1.,0.,0.));
#9599=DIRECTION('ref_axis',(0.,-1.,0.));
#9600=DIRECTION('center_axis',(0.,1.,-2.79713066068216E-16));
#9601=DIRECTION('ref_axis',(0.,2.79713066068216E-16,1.));
#9602=DIRECTION('',(1.,0.,0.));
#9603=DIRECTION('center_axis',(1.,0.,0.));
#9604=DIRECTION('ref_axis',(0.,-1.,0.));
#9605=DIRECTION('center_axis',(1.,0.,0.));
#9606=DIRECTION('ref_axis',(0.,-1.,0.));
#9607=DIRECTION('',(1.,0.,0.));
#9608=DIRECTION('center_axis',(-1.,0.,0.));
#9609=DIRECTION('ref_axis',(0.,0.,1.));
#9610=DIRECTION('center_axis',(-1.,0.,0.));
#9611=DIRECTION('ref_axis',(0.,0.,1.));
#9612=DIRECTION('',(-1.,0.,0.));
#9613=DIRECTION('center_axis',(0.,0.,-1.));
#9614=DIRECTION('ref_axis',(0.,-1.,0.));
#9615=DIRECTION('',(-1.,0.,0.));
#9616=DIRECTION('center_axis',(0.,0.,-1.));
#9617=DIRECTION('ref_axis',(0.,-1.,0.));
#9618=DIRECTION('',(0.,-1.,0.));
#9619=DIRECTION('',(1.,0.,0.));
#9620=DIRECTION('center_axis',(1.,0.,0.));
#9621=DIRECTION('ref_axis',(0.,1.,0.));
#9622=DIRECTION('',(0.,0.,-1.));
#9623=DIRECTION('center_axis',(0.,1.,0.));
#9624=DIRECTION('ref_axis',(0.,0.,1.));
#9625=DIRECTION('',(1.,0.,0.));
#9626=DIRECTION('center_axis',(-1.,0.,0.));
#9627=DIRECTION('ref_axis',(0.,0.,-1.));
#9628=DIRECTION('center_axis',(0.,0.,1.));
#9629=DIRECTION('ref_axis',(0.,1.,0.));
#9630=DIRECTION('',(-1.,0.,0.));
#9631=DIRECTION('',(0.,1.,0.));
#9632=DIRECTION('center_axis',(0.,1.,0.));
#9633=DIRECTION('ref_axis',(0.,0.,-1.));
#9634=DIRECTION('',(0.,0.,-1.));
#9635=DIRECTION('',(-1.,0.,0.));
#9636=DIRECTION('center_axis',(-1.,0.,0.));
#9637=DIRECTION('ref_axis',(0.,1.,0.));
#9638=DIRECTION('center_axis',(-1.,0.,0.));
#9639=DIRECTION('ref_axis',(0.,1.,0.));
#9640=DIRECTION('center_axis',(1.,0.,0.));
#9641=DIRECTION('ref_axis',(0.,1.,0.));
#9642=DIRECTION('center_axis',(0.,0.,1.));
#9643=DIRECTION('ref_axis',(0.,1.,0.));
#9644=DIRECTION('center_axis',(0.,1.,0.));
#9645=DIRECTION('ref_axis',(0.707106781186549,0.,-0.707106781186546));
#9646=DIRECTION('center_axis',(0.,1.,0.));
#9647=DIRECTION('ref_axis',(1.,0.,0.));
#9648=DIRECTION('',(0.,1.,0.));
#9649=DIRECTION('center_axis',(0.,-1.,0.));
#9650=DIRECTION('ref_axis',(0.,0.,-1.));
#9651=DIRECTION('center_axis',(-1.,0.,0.));
#9652=DIRECTION('ref_axis',(0.,0.,1.));
#9653=DIRECTION('center_axis',(0.,1.,0.));
#9654=DIRECTION('ref_axis',(0.,0.,1.));
#9655=DIRECTION('center_axis',(-1.,0.,0.));
#9656=DIRECTION('ref_axis',(0.,1.,0.));
#9657=DIRECTION('center_axis',(0.,-1.,0.));
#9658=DIRECTION('ref_axis',(0.707106781186549,0.,0.707106781186546));
#9659=DIRECTION('center_axis',(0.,1.,0.));
#9660=DIRECTION('ref_axis',(0.,0.,1.));
#9661=DIRECTION('',(0.,-1.,0.));
#9662=DIRECTION('center_axis',(-1.,0.,0.));
#9663=DIRECTION('ref_axis',(0.,0.,1.));
#9664=DIRECTION('center_axis',(0.,-0.96848146623447,0.249085626964569));
#9665=DIRECTION('ref_axis',(1.,0.,0.));
#9666=DIRECTION('center_axis',(-1.,0.,0.));
#9667=DIRECTION('ref_axis',(0.,-0.790280212002226,-0.612745613217848));
#9668=DIRECTION('center_axis',(0.,0.,-1.));
#9669=DIRECTION('ref_axis',(0.,1.,0.));
#9670=DIRECTION('center_axis',(0.,2.79713066068216E-16,1.));
#9671=DIRECTION('ref_axis',(0.707106781186546,0.707106781186549,0.));
#9672=DIRECTION('center_axis',(0.,0.,-1.));
#9673=DIRECTION('ref_axis',(0.,1.,0.));
#9674=DIRECTION('',(0.,2.79713066068216E-16,1.));
#9675=DIRECTION('center_axis',(0.,1.,0.));
#9676=DIRECTION('ref_axis',(0.,0.,1.));
#9677=DIRECTION('center_axis',(1.,0.,0.));
#9678=DIRECTION('ref_axis',(0.,0.707106781186548,0.707106781186547));
#9679=DIRECTION('center_axis',(0.,-1.,0.));
#9680=DIRECTION('ref_axis',(0.707106781186549,0.,0.707106781186546));
#9681=DIRECTION('center_axis',(0.,1.,0.));
#9682=DIRECTION('ref_axis',(0.,0.,1.));
#9683=DIRECTION('center_axis',(0.,0.,1.));
#9684=DIRECTION('ref_axis',(0.,-1.,0.));
#9685=DIRECTION('center_axis',(1.,0.,0.));
#9686=DIRECTION('ref_axis',(0.,-0.707106781186549,0.707106781186546));
#9687=DIRECTION('center_axis',(0.,0.,-1.));
#9688=DIRECTION('ref_axis',(0.707106781186548,-0.707106781186548,0.));
#9689=DIRECTION('center_axis',(0.,0.,1.));
#9690=DIRECTION('ref_axis',(0.,-1.,0.));
#9691=DIRECTION('center_axis',(0.,-1.,0.));
#9692=DIRECTION('ref_axis',(0.707106781186549,0.,0.707106781186546));
#9693=DIRECTION('center_axis',(0.,-1.,0.));
#9694=DIRECTION('ref_axis',(1.,0.,0.));
#9695=DIRECTION('',(0.,-1.,0.));
#9696=DIRECTION('center_axis',(0.,1.,0.));
#9697=DIRECTION('ref_axis',(0.,0.,1.));
#9698=DIRECTION('center_axis',(-1.,0.,0.));
#9699=DIRECTION('ref_axis',(0.,0.,1.));
#9700=DIRECTION('center_axis',(0.,-0.435505427952634,-0.900186104216119));
#9701=DIRECTION('ref_axis',(0.,0.900186104216119,-0.435505427952634));
#9702=DIRECTION('center_axis',(-1.,0.,0.));
#9703=DIRECTION('ref_axis',(0.,-0.847202876515606,-0.531269504134844));
#9704=DIRECTION('center_axis',(-0.816496580927726,0.408248290463863,0.408248290463863));
#9705=DIRECTION('ref_axis',(0.577350269189628,0.577350269189627,0.577350269189623));
#9706=DIRECTION('center_axis',(1.,0.,0.));
#9707=DIRECTION('ref_axis',(0.,0.707106781186548,0.707106781186548));
#9708=DIRECTION('center_axis',(0.,0.,1.));
#9709=DIRECTION('ref_axis',(1.,0.,0.));
#9710=DIRECTION('center_axis',(1.,0.,0.));
#9711=DIRECTION('ref_axis',(0.,-0.249085626964568,-0.96848146623447));
#9712=DIRECTION('center_axis',(-0.816496580927726,-0.408248290463865,-0.40824829046386));
#9713=DIRECTION('ref_axis',(0.577350269189627,-0.577350269189627,-0.577350269189623));
#9714=DIRECTION('center_axis',(1.,0.,0.));
#9715=DIRECTION('ref_axis',(0.,-0.707106781186549,-0.707106781186546));
#9716=DIRECTION('center_axis',(-0.816496580927725,-0.408248290463865,0.408248290463863));
#9717=DIRECTION('ref_axis',(0.577350269189627,-0.577350269189627,0.577350269189623));
#9718=DIRECTION('center_axis',(1.,0.,0.));
#9719=DIRECTION('ref_axis',(0.,-0.707106781186549,0.707106781186546));
#9720=DIRECTION('center_axis',(-1.,0.,0.));
#9721=DIRECTION('ref_axis',(0.,-0.707106781186549,0.707106781186546));
#9722=DIRECTION('',(-1.,0.,0.));
#9723=DIRECTION('center_axis',(-1.,0.,0.));
#9724=DIRECTION('ref_axis',(0.,-0.707106781186549,0.707106781186546));
#9725=DIRECTION('center_axis',(0.,0.,-1.));
#9726=DIRECTION('ref_axis',(0.,-1.,0.));
#9727=DIRECTION('',(-1.,0.,0.));
#9728=DIRECTION('',(0.,-1.,0.));
#9729=DIRECTION('center_axis',(-1.,0.,0.));
#9730=DIRECTION('ref_axis',(0.,0.,-1.));
#9731=DIRECTION('',(-1.,0.,0.));
#9732=DIRECTION('center_axis',(-1.,0.,0.));
#9733=DIRECTION('ref_axis',(0.,0.,-1.));
#9734=DIRECTION('center_axis',(0.,0.,1.));
#9735=DIRECTION('ref_axis',(0.,1.,0.));
#9736=DIRECTION('',(1.,0.,0.));
#9737=DIRECTION('',(0.,1.,0.));
#9738=DIRECTION('center_axis',(1.,0.,0.));
#9739=DIRECTION('ref_axis',(0.,-0.707106781186549,-0.707106781186546));
#9740=DIRECTION('center_axis',(-1.,0.,0.));
#9741=DIRECTION('ref_axis',(0.,-0.707106781186549,-0.707106781186546));
#9742=DIRECTION('center_axis',(1.,0.,0.));
#9743=DIRECTION('ref_axis',(0.,-0.707106781186549,0.707106781186546));
#9744=DIRECTION('center_axis',(1.,0.,0.));
#9745=DIRECTION('ref_axis',(0.,0.707106781186548,0.707106781186547));
#9746=DIRECTION('',(-1.,0.,0.));
#9747=DIRECTION('center_axis',(0.,1.,-2.79713066068216E-16));
#9748=DIRECTION('ref_axis',(0.,2.79713066068216E-16,1.));
#9749=DIRECTION('',(1.,0.,0.));
#9750=DIRECTION('center_axis',(1.,0.,0.));
#9751=DIRECTION('ref_axis',(0.,-1.,0.));
#9752=DIRECTION('',(1.,0.,0.));
#9753=DIRECTION('center_axis',(-1.,0.,0.));
#9754=DIRECTION('ref_axis',(0.,-1.,0.));
#9755=DIRECTION('',(1.,0.,0.));
#9756=DIRECTION('center_axis',(-1.,0.,0.));
#9757=DIRECTION('ref_axis',(0.,-0.249085626964568,-0.96848146623447));
#9758=DIRECTION('',(-1.,0.,0.));
#9759=DIRECTION('center_axis',(-1.,0.,0.));
#9760=DIRECTION('ref_axis',(0.,-0.249085626964568,-0.96848146623447));
#9761=DIRECTION('center_axis',(-1.,0.,0.));
#9762=DIRECTION('ref_axis',(0.,0.,1.));
#9763=DIRECTION('',(-1.,0.,0.));
#9764=DIRECTION('center_axis',(-1.,0.,0.));
#9765=DIRECTION('ref_axis',(0.,0.,1.));
#9766=DIRECTION('center_axis',(0.,0.,-1.));
#9767=DIRECTION('ref_axis',(0.,-1.,0.));
#9768=DIRECTION('',(1.,0.,0.));
#9769=DIRECTION('',(0.,-1.,0.));
#9770=DIRECTION('center_axis',(1.,0.,0.));
#9771=DIRECTION('ref_axis',(0.,0.707106781186548,0.707106781186548));
#9772=DIRECTION('center_axis',(-1.,0.,0.));
#9773=DIRECTION('ref_axis',(0.,0.707106781186548,0.707106781186548));
#9774=DIRECTION('center_axis',(0.,0.,1.));
#9775=DIRECTION('ref_axis',(0.,1.,0.));
#9776=DIRECTION('',(0.,1.,0.));
#9777=DIRECTION('',(-1.,0.,0.));
#9778=DIRECTION('center_axis',(0.,1.,0.));
#9779=DIRECTION('ref_axis',(0.,0.,-1.));
#9780=DIRECTION('',(-1.,0.,0.));
#9781=DIRECTION('',(0.,0.,-1.));
#9782=DIRECTION('',(-1.,0.,0.));
#9783=DIRECTION('center_axis',(-1.,0.,0.));
#9784=DIRECTION('ref_axis',(0.,1.,0.));
#9785=DIRECTION('center_axis',(-1.,0.,0.));
#9786=DIRECTION('ref_axis',(0.,1.,0.));
#9787=DIRECTION('center_axis',(1.,0.,0.));
#9788=DIRECTION('ref_axis',(0.,1.,0.));
#9789=DIRECTION('center_axis',(-1.,0.,0.));
#9790=DIRECTION('ref_axis',(0.,-1.,0.));
#9791=DIRECTION('',(0.,-1.,0.));
#9792=DIRECTION('center_axis',(1.,0.,0.));
#9793=DIRECTION('ref_axis',(0.,1.,0.));
#9794=DIRECTION('',(0.,-1.,0.));
#9795=DIRECTION('center_axis',(-1.,0.,0.));
#9796=DIRECTION('ref_axis',(0.,1.,-4.44089209850062E-15));
#9797=DIRECTION('center_axis',(0.,0.,1.));
#9798=DIRECTION('ref_axis',(0.,1.,0.));
#9799=DIRECTION('',(-1.,0.,0.));
#9800=DIRECTION('',(0.,1.,0.));
#9801=DIRECTION('center_axis',(-1.,0.,0.));
#9802=DIRECTION('ref_axis',(0.,0.,1.));
#9803=DIRECTION('',(-1.,0.,0.));
#9804=DIRECTION('center_axis',(-1.,0.,0.));
#9805=DIRECTION('ref_axis',(0.,0.,1.));
#9806=DIRECTION('center_axis',(0.,-1.,0.));
#9807=DIRECTION('ref_axis',(0.,0.,1.));
#9808=DIRECTION('',(1.,0.,0.));
#9809=DIRECTION('',(0.,0.,1.));
#9810=DIRECTION('center_axis',(1.,0.,0.));
#9811=DIRECTION('ref_axis',(0.,1.,0.));
#9812=DIRECTION('',(0.,-1.,0.));
#9813=DIRECTION('center_axis',(-1.,0.,0.));
#9814=DIRECTION('ref_axis',(0.,-1.11022302462516E-15,-1.));
#9815=DIRECTION('center_axis',(1.,0.,0.));
#9816=DIRECTION('ref_axis',(0.,1.,0.));
#9817=DIRECTION('center_axis',(0.,0.,1.));
#9818=DIRECTION('ref_axis',(0.,-1.,0.));
#9819=DIRECTION('',(1.,0.,0.));
#9820=DIRECTION('center_axis',(0.,0.,-1.));
#9821=DIRECTION('ref_axis',(0.,1.,0.));
#9822=DIRECTION('',(1.,0.,0.));
#9823=DIRECTION('',(1.,0.,0.));
#9824=DIRECTION('center_axis',(1.,0.,0.));
#9825=DIRECTION('ref_axis',(0.,1.,-4.44089209850062E-15));
#9826=DIRECTION('center_axis',(1.,0.,0.));
#9827=DIRECTION('ref_axis',(0.,-1.11022302462516E-15,-1.));
#9828=DIRECTION('center_axis',(1.,0.,0.));
#9829=DIRECTION('ref_axis',(0.,-1.,0.));
#11812=CARTESIAN_POINT('',(0.,0.,0.));
#11813=CARTESIAN_POINT('Origin',(8.5,25.0098518119976,-22.4105093470644));
#11814=CARTESIAN_POINT('',(0.499999999999999,22.2688065021356,-18.8416621089099));
#11815=CARTESIAN_POINT('',(1.74028546827764,22.2688065021356,-18.8416621089099));
#11816=CARTESIAN_POINT('',(8.5,22.2688065021356,-18.8416621089099));
#11817=CARTESIAN_POINT('',(2.74028546827765,21.2688065021356,-19.9095935169016));
#11818=CARTESIAN_POINT('Ctrl Pts',(1.74028546827765,22.2688065021356,-18.8416621089099));
#11819=CARTESIAN_POINT('Ctrl Pts',(1.83421821452936,22.2688065021356,-18.8416621089099));
#11820=CARTESIAN_POINT('Ctrl Pts',(1.93470401993251,22.2546061414744,-18.8524321964904));
#11821=CARTESIAN_POINT('Ctrl Pts',(2.12234108686958,22.1981250134701,-18.8968952198158));
#11822=CARTESIAN_POINT('Ctrl Pts',(2.20951967834708,22.1560062467128,-18.9306784121546));
#11823=CARTESIAN_POINT('Ctrl Pts',(2.38012940236584,22.0462287372975,-19.0232033412094));
#11824=CARTESIAN_POINT('Ctrl Pts',(2.46708450855627,21.9643664133557,-19.0954331993668));
#11825=CARTESIAN_POINT('Ctrl Pts',(2.60062014887845,21.7902127170047,-19.2642996258922));
#11826=CARTESIAN_POINT('Ctrl Pts',(2.64760861619124,21.6983105804248,-19.361014553391));
#11827=CARTESIAN_POINT('Ctrl Pts',(2.72401108672779,21.4919221323301,-19.5980623673013));
#11828=CARTESIAN_POINT('Ctrl Pts',(2.74028546827765,21.3756357329717,-19.7497908605485));
#11829=CARTESIAN_POINT('Ctrl Pts',(2.74028546827765,21.2688065021356,-19.9095935169016));
#11830=CARTESIAN_POINT('',(2.74028546827765,20.5098518119976,-22.4105093470644));
#11831=CARTESIAN_POINT('Origin',(2.74028546827764,25.0098518119976,-22.4105093470644));
#11832=CARTESIAN_POINT('',(6.5,20.5098518119976,-22.4105093470644));
#11833=CARTESIAN_POINT('',(8.5,20.5098518119976,-22.4105093470644));
#11834=CARTESIAN_POINT('',(6.5,25.0098518119976,-17.9105093470644));
#11835=CARTESIAN_POINT('Origin',(6.5,25.0098518119976,-22.4105093470644));
#11836=CARTESIAN_POINT('',(0.499999999999999,25.0098518119976,-17.9105093470644));
#11837=CARTESIAN_POINT('',(8.5,25.0098518119976,-17.9105093470644));
#11838=CARTESIAN_POINT('Origin',(0.499999999999999,25.0098518119976,-22.4105093470644));
#11839=CARTESIAN_POINT('Origin',(8.5,20.5098518119976,-25.0483789742253));
#11840=CARTESIAN_POINT('',(2.74028546827764,20.5098518119976,-23.0483789742253));
#11841=CARTESIAN_POINT('',(2.74028546827765,20.5098518119976,-25.0483789742253));
#11842=CARTESIAN_POINT('',(6.5,20.5098518119976,-23.0483789742253));
#11843=CARTESIAN_POINT('',(1.,20.5098518119976,-23.0483789742253));
#11844=CARTESIAN_POINT('',(6.5,20.5098518119976,-6.56473183187052));
#11845=CARTESIAN_POINT('Origin',(1.74028546827764,22.2688065021356,-25.0483789742253));
#11846=CARTESIAN_POINT('',(-0.5,22.2688065021356,-25.0483789742253));
#11847=CARTESIAN_POINT('',(-0.5,22.2688065021356,-23.0483789742253));
#11848=CARTESIAN_POINT('',(-0.499999999999999,22.2688065021356,-6.56473183187052));
#11849=CARTESIAN_POINT('',(1.74028546827764,22.2688065021356,-25.0483789742253));
#11850=CARTESIAN_POINT('',(-2.37985726586118,22.2688065021356,-25.0483789742253));
#11851=CARTESIAN_POINT('',(1.74028546827764,22.2688065021356,-25.0483789742253));
#11852=CARTESIAN_POINT('',(0.5,22.2688065021356,-23.0483789742253));
#11853=CARTESIAN_POINT('',(0.499999999999999,22.2688065021356,-23.7639115674351));
#11854=CARTESIAN_POINT('',(-2.37985726586118,22.2688065021356,-23.0483789742253));
#11855=CARTESIAN_POINT('Origin',(1.74028546827765,21.2688065021356,-25.0483789742253));
#11856=CARTESIAN_POINT('',(2.74028546827765,21.2688065021356,-25.0483789742253));
#11857=CARTESIAN_POINT('Origin',(1.74028546827765,21.2688065021356,-25.0483789742253));
#11858=CARTESIAN_POINT('',(2.74028546827765,21.2688065021356,-25.0483789742253));
#11859=CARTESIAN_POINT('Origin',(2.74028546827764,17.8031073387245,-25.0483789742253));
#11860=CARTESIAN_POINT('',(2.74028546827764,17.8031073387245,-25.0483789742253));
#11861=CARTESIAN_POINT('',(2.74028546827764,5.68566717807833,-25.0483789742253));
#11862=CARTESIAN_POINT('',(2.74028546827764,17.8031073387245,-23.0483789742253));
#11863=CARTESIAN_POINT('',(2.74028546827764,17.8031073387245,-25.0483789742253));
#11864=CARTESIAN_POINT('',(2.74028546827764,5.68566717807833,-23.0483789742253));
#11865=CARTESIAN_POINT('Origin',(1.74028546827765,17.8031073387245,-25.0483789742253));
#11866=CARTESIAN_POINT('',(1.74028546827765,16.8031073387245,-25.0483789742253));
#11867=CARTESIAN_POINT('Origin',(1.74028546827765,17.8031073387245,-25.0483789742253));
#11868=CARTESIAN_POINT('',(1.74028546827765,16.8031073387245,-23.0483789742253));
#11869=CARTESIAN_POINT('',(1.74028546827765,16.8031073387245,-25.0483789742253));
#11870=CARTESIAN_POINT('Origin',(1.74028546827765,17.8031073387245,-23.0483789742253));
#11871=CARTESIAN_POINT('Origin',(-14.7402854682776,16.8031073387245,-25.0483789742253));
#11872=CARTESIAN_POINT('',(-0.499999999999999,16.8031073387245,-23.0483789742253));
#11873=CARTESIAN_POINT('',(-0.499999999999999,16.8031073387245,-25.0483789742253));
#11874=CARTESIAN_POINT('',(-0.499999999999999,16.8031073387245,-6.56473183187052));
#11875=CARTESIAN_POINT('',(-10.6201427341388,16.8031073387245,-23.0483789742253));
#11876=CARTESIAN_POINT('',(-10.6201427341388,16.8031073387245,-25.0483789742253));
#11877=CARTESIAN_POINT('Origin',(-6.5,-6.43177298256785,-23.0483789742253));
#11878=CARTESIAN_POINT('',(0.499999999999999,23.6522353938789,-23.0483789742253));
#11879=CARTESIAN_POINT('',(0.499999999999999,9.27063275147817,-23.0483789742253));
#11880=CARTESIAN_POINT('',(-0.499999999999999,23.6522353938789,-23.0483789742253));
#11881=CARTESIAN_POINT('',(8.5,23.6522353938789,-23.0483789742253));
#11882=CARTESIAN_POINT('',(-0.499999999999999,1.53522655283679,-23.0483789742253));
#11883=CARTESIAN_POINT('Origin',(-6.5,-6.43177298256785,-23.0483789742253));
#11884=CARTESIAN_POINT('',(-0.499999999999999,-4.64778321739598,-23.0483789742253));
#11885=CARTESIAN_POINT('',(-0.499999999999999,1.53522655283679,-23.0483789742253));
#11886=CARTESIAN_POINT('',(0.499999999999999,-4.64778321739598,-23.0483789742253));
#11887=CARTESIAN_POINT('',(8.5,-4.64778321739598,-23.0483789742253));
#11888=CARTESIAN_POINT('',(0.499999999999998,-1.50539963551477,-23.0483789742253));
#11889=CARTESIAN_POINT('',(0.499999999999999,-6.20017964580458,-23.0483789742253));
#11890=CARTESIAN_POINT('',(6.5,-1.50539963551477,-23.0483789742253));
#11891=CARTESIAN_POINT('',(1.,-1.50539963551477,-23.0483789742253));
#11892=CARTESIAN_POINT('',(6.5,1.53522655283679,-23.0483789742253));
#11893=CARTESIAN_POINT('Origin',(-0.499999999999999,9.50222608824143,11.9189153104842));
#11894=CARTESIAN_POINT('',(-0.499999999999999,-6.43177298256785,-25.0483789742253));
#11895=CARTESIAN_POINT('',(-0.499999999999999,1.53522655283679,-25.0483789742253));
#11896=CARTESIAN_POINT('',(-0.499999999999999,-8.43177298256785,-23.0483789742253));
#11897=CARTESIAN_POINT('Origin',(-0.499999999999999,-6.43177298256785,-23.0483789742253));
#11898=CARTESIAN_POINT('',(-0.499999999999999,-8.43177298256785,46.8862095951938));
#11899=CARTESIAN_POINT('',(-0.499999999999999,-8.43177298256785,30.402562452839));
#11900=CARTESIAN_POINT('',(-0.499999999999999,-6.43177298256785,48.8862095951938));
#11901=CARTESIAN_POINT('Origin',(-0.499999999999999,-6.43177298256785,46.8862095951938));
#11902=CARTESIAN_POINT('',(-0.499999999999999,-5.56822701743215,48.8862095951938));
#11903=CARTESIAN_POINT('',(-0.499999999999999,2.03522655283679,48.8862095951938));
#11904=CARTESIAN_POINT('',(-0.499999999999999,-5.56822701743215,46.8862095951938));
#11905=CARTESIAN_POINT('',(-0.499999999999999,-5.56822701743215,30.402562452839));
#11906=CARTESIAN_POINT('',(-0.499999999999999,-6.43177298256785,46.8862095951938));
#11907=CARTESIAN_POINT('',(-0.499999999999999,15.3987725179725,46.8862095951938));
#11908=CARTESIAN_POINT('',(-0.499999999999999,-6.43177298256785,30.9666314003931));
#11909=CARTESIAN_POINT('',(-0.499999999999999,-6.43177298256785,30.402562452839));
#11910=CARTESIAN_POINT('',(-0.499999999999999,-7.44334688204796,29.5483789742253));
#11911=CARTESIAN_POINT('Origin',(-0.499999999999999,-5.94334688204796,29.5483789742253));
#11912=CARTESIAN_POINT('',(-0.499999999999999,-6.43177298256785,28.1301265480575));
#11913=CARTESIAN_POINT('Origin',(-0.499999999999999,-5.94334688204796,29.5483789742253));
#11914=CARTESIAN_POINT('',(-0.499999999999999,-6.43177298256785,-20.9723835636495));
#11915=CARTESIAN_POINT('',(-0.499999999999999,-6.43177298256785,30.402562452839));
#11916=CARTESIAN_POINT('',(-0.499999999999999,-7.50539963551477,-22.4105093470644));
#11917=CARTESIAN_POINT('Origin',(-0.499999999999999,-6.00539963551477,-22.4105093470644));
#11918=CARTESIAN_POINT('Origin',(-0.499999999999999,-6.00539963551477,-22.4105093470644));
#11919=CARTESIAN_POINT('Origin',(1.,-7.43177298256785,-18.9105093470644));
#11920=CARTESIAN_POINT('',(7.5,-7.43177298256785,-19.9105093470644));
#11921=CARTESIAN_POINT('',(7.5,-8.43177298256785,-18.9105093470644));
#11922=CARTESIAN_POINT('Origin',(7.5,-7.43177298256785,-18.9105093470644));
#11923=CARTESIAN_POINT('',(2.5,-8.43177298256785,-18.9105093470644));
#11924=CARTESIAN_POINT('',(1.,-8.43177298256785,-18.9105093470644));
#11925=CARTESIAN_POINT('',(2.5,-7.43177298256785,-19.9105093470644));
#11926=CARTESIAN_POINT('Origin',(2.5,-7.43177298256785,-18.9105093470644));
#11927=CARTESIAN_POINT('',(1.,-7.43177298256785,-19.9105093470644));
#11928=CARTESIAN_POINT('Origin',(7.5,21.5098518119976,-6.56473183187052));
#11929=CARTESIAN_POINT('',(7.5,22.5098518119976,-25.0483789742253));
#11930=CARTESIAN_POINT('',(7.5,22.5098518119976,-22.4105093470644));
#11931=CARTESIAN_POINT('',(7.5,22.5098518119976,-6.56473183187052));
#11932=CARTESIAN_POINT('',(8.5,21.5098518119976,-22.4105093470644));
#11933=CARTESIAN_POINT('Origin',(7.5,21.5098518119976,-22.4105093470644));
#11934=CARTESIAN_POINT('',(8.5,21.5098518119976,-24.0483789742253));
#11935=CARTESIAN_POINT('',(8.5,21.5098518119976,-6.56473183187052));
#11936=CARTESIAN_POINT('Origin',(7.5,21.5098518119976,-24.0483789742253));
#11937=CARTESIAN_POINT('Origin',(7.5,1.53522655283679,-24.0483789742253));
#11938=CARTESIAN_POINT('',(8.5,-2.50539963551477,-24.0483789742253));
#11939=CARTESIAN_POINT('',(8.5,1.53522655283679,-24.0483789742253));
#11940=CARTESIAN_POINT('',(7.5,-3.50539963551477,-25.0483789742253));
#11941=CARTESIAN_POINT('Origin',(7.5,-2.50539963551477,-24.0483789742253));
#11942=CARTESIAN_POINT('',(7.5,1.53522655283679,-25.0483789742253));
#11943=CARTESIAN_POINT('Origin',(7.5,0.535226552836792,-18.9105093470644));
#11944=CARTESIAN_POINT('',(8.5,-7.43177298256785,-18.9105093470644));
#11945=CARTESIAN_POINT('Origin',(7.5,-7.43177298256785,-18.9105093470644));
#11946=CARTESIAN_POINT('',(7.5,-6.00539963551477,-19.9105093470644));
#11947=CARTESIAN_POINT('',(7.5,0.535226552836792,-19.9105093470644));
#11948=CARTESIAN_POINT('',(8.5,-6.00539963551477,-18.9105093470644));
#11949=CARTESIAN_POINT('Origin',(7.5,-6.00539963551477,-18.9105093470644));
#11950=CARTESIAN_POINT('',(8.5,0.535226552836792,-18.9105093470644));
#11951=CARTESIAN_POINT('Origin',(7.5,-6.00539963551477,-22.4105093470644));
#11952=CARTESIAN_POINT('',(7.5,-3.50539963551477,-22.4105093470644));
#11953=CARTESIAN_POINT('',(8.5,-2.50539963551477,-22.4105093470644));
#11954=CARTESIAN_POINT('Origin',(7.5,-2.50539963551477,-22.4105093470644));
#11955=CARTESIAN_POINT('Origin',(8.5,-6.00539963551477,-22.4105093470644));
#11956=CARTESIAN_POINT('Origin',(7.5,-6.00539963551477,-22.4105093470644));
#11957=CARTESIAN_POINT('Origin',(7.5,-2.50539963551477,-5.2457970182901));
#11958=CARTESIAN_POINT('',(8.5,-2.50539963551477,-5.2457970182901));
#11959=CARTESIAN_POINT('',(7.5,-3.50539963551477,-5.2457970182901));
#11960=CARTESIAN_POINT('Origin',(7.5,25.0098518119976,-22.4105093470644));
#11961=CARTESIAN_POINT('',(7.5,25.0098518119976,-19.9105093470644));
#11962=CARTESIAN_POINT('',(8.5,25.0098518119976,-18.9105093470644));
#11963=CARTESIAN_POINT('Origin',(7.5,25.0098518119976,-18.9105093470644));
#11964=CARTESIAN_POINT('Origin',(8.5,25.0098518119976,-22.4105093470644));
#11965=CARTESIAN_POINT('Origin',(7.5,25.0098518119976,-22.4105093470644));
#11966=CARTESIAN_POINT('Origin',(7.5,17.2560389501195,-18.9105093470644));
#11967=CARTESIAN_POINT('',(7.5,26.4362251590507,-19.9105093470644));
#11968=CARTESIAN_POINT('',(8.5,26.4362251590507,-18.9105093470644));
#11969=CARTESIAN_POINT('Origin',(7.5,26.4362251590507,-18.9105093470644));
#11970=CARTESIAN_POINT('',(8.5,17.2560389501195,-18.9105093470644));
#11971=CARTESIAN_POINT('',(7.5,17.2560389501195,-19.9105093470644));
#11972=CARTESIAN_POINT('Origin',(7.5,-7.43177298256785,-18.9105093470644));
#11973=CARTESIAN_POINT('Origin',(7.5,-7.43177298256785,-18.9105093470644));
#11974=CARTESIAN_POINT('Origin',(1.,26.4362251590507,-18.9105093470644));
#11975=CARTESIAN_POINT('',(7.5,27.4362251590507,-18.9105093470644));
#11976=CARTESIAN_POINT('Origin',(7.5,26.4362251590507,-18.9105093470644));
#11977=CARTESIAN_POINT('',(2.5,26.4362251590507,-19.9105093470644));
#11978=CARTESIAN_POINT('',(1.,26.4362251590507,-19.9105093470644));
#11979=CARTESIAN_POINT('',(2.5,27.4362251590507,-18.9105093470644));
#11980=CARTESIAN_POINT('Origin',(2.5,26.4362251590507,-18.9105093470644));
#11981=CARTESIAN_POINT('',(1.,27.4362251590507,-18.9105093470644));
#11982=CARTESIAN_POINT('Origin',(7.5,26.4362251590507,-18.9105093470644));
#11983=CARTESIAN_POINT('Origin',(7.5,26.4362251590507,-18.9105093470644));
#11984=CARTESIAN_POINT('Origin',(-6.5,-8.43177298256785,48.8862095951938));
#11985=CARTESIAN_POINT('',(2.5,-8.43177298256785,-23.0483789742253));
#11986=CARTESIAN_POINT('',(2.5,-8.43177298256785,13.2033827172745));
#11987=CARTESIAN_POINT('',(7.5,-8.43177298256785,26.0483789742253));
#11988=CARTESIAN_POINT('',(7.5,-8.43177298256785,30.402562452839));
#11989=CARTESIAN_POINT('',(2.5,-8.43177298256785,26.0483789742253));
#11990=CARTESIAN_POINT('',(1.,-8.43177298256785,26.0483789742253));
#11991=CARTESIAN_POINT('',(2.5,-8.43177298256785,33.0483789742253));
#11992=CARTESIAN_POINT('',(2.5,-8.43177298256785,39.2172942847095));
#11993=CARTESIAN_POINT('',(7.5,-8.43177298256785,33.0483789742253));
#11994=CARTESIAN_POINT('',(1.,-8.43177298256785,33.0483789742253));
#11995=CARTESIAN_POINT('',(7.5,-8.43177298256785,46.8862095951938));
#11996=CARTESIAN_POINT('',(7.5,-8.43177298256785,30.402562452839));
#11997=CARTESIAN_POINT('',(-6.5,-8.43177298256785,46.8862095951938));
#11998=CARTESIAN_POINT('',(-6.5,-8.43177298256785,-23.0483789742253));
#11999=CARTESIAN_POINT('Origin',(7.5,-7.43177298256785,30.402562452839));
#12000=CARTESIAN_POINT('',(8.5,-7.43177298256785,26.0483789742253));
#12001=CARTESIAN_POINT('',(8.5,-7.43177298256785,30.402562452839));
#12002=CARTESIAN_POINT('Origin',(7.5,-7.43177298256785,26.0483789742253));
#12003=CARTESIAN_POINT('Origin',(8.5,9.50222608824143,11.9189153104842));
#12004=CARTESIAN_POINT('',(8.5,26.4362251590507,26.0483789742253));
#12005=CARTESIAN_POINT('',(8.5,26.4362251590507,-5.56473183187052));
#12006=CARTESIAN_POINT('',(8.5,24.9477990585308,26.0483789742253));
#12007=CARTESIAN_POINT('',(8.5,18.4692256236461,26.0483789742253));
#12008=CARTESIAN_POINT('',(8.5,21.7971476937744,31.0726479720595));
#12009=CARTESIAN_POINT('Origin',(8.5,24.9477990585308,29.5483789742253));
#12010=CARTESIAN_POINT('',(8.5,20.2953189477035,33.0096109045284));
#12011=CARTESIAN_POINT('Origin',(8.5,22.2953189477035,33.0096109045284));
#12012=CARTESIAN_POINT('',(8.5,20.2953189477035,46.8862095951938));
#12013=CARTESIAN_POINT('',(8.5,20.2953189477035,22.4642631075063));
#12014=CARTESIAN_POINT('',(8.5,19.2953189477036,47.8862095951938));
#12015=CARTESIAN_POINT('Origin',(8.5,19.2953189477036,46.8862095951938));
#12016=CARTESIAN_POINT('',(8.5,-6.43177298256785,47.8862095951938));
#12017=CARTESIAN_POINT('',(8.5,15.3987725179725,47.8862095951938));
#12018=CARTESIAN_POINT('',(8.5,-7.43177298256785,46.8862095951938));
#12019=CARTESIAN_POINT('Origin',(8.5,-6.43177298256785,46.8862095951938));
#12020=CARTESIAN_POINT('',(8.5,-7.43177298256785,33.0483789742253));
#12021=CARTESIAN_POINT('',(8.5,-7.43177298256785,30.402562452839));
#12022=CARTESIAN_POINT('',(8.5,-5.94334688204796,33.0483789742253));
#12023=CARTESIAN_POINT('',(8.5,0.535226552836791,33.0483789742253));
#12024=CARTESIAN_POINT('',(8.5,-5.94334688204796,26.0483789742253));
#12025=CARTESIAN_POINT('Origin',(8.5,-5.94334688204796,29.5483789742253));
#12026=CARTESIAN_POINT('',(8.5,1.77943960309674,26.0483789742253));
#12027=CARTESIAN_POINT('Origin',(7.5,26.4362251590507,-5.56473183187052));
#12028=CARTESIAN_POINT('',(7.5,27.4362251590507,26.0483789742253));
#12029=CARTESIAN_POINT('',(7.5,27.4362251590507,-5.56473183187052));
#12030=CARTESIAN_POINT('Origin',(7.5,26.4362251590507,26.0483789742253));
#12031=CARTESIAN_POINT('Origin',(-6.5,27.4362251590507,-23.0483789742253));
#12032=CARTESIAN_POINT('',(2.5,27.4362251590507,-23.0483789742253));
#12033=CARTESIAN_POINT('',(2.5,27.4362251590507,-22.7639115674351));
#12034=CARTESIAN_POINT('',(-0.499999999999999,27.4362251590507,-23.0483789742253));
#12035=CARTESIAN_POINT('',(-6.5,27.4362251590507,-23.0483789742253));
#12036=CARTESIAN_POINT('',(-0.499999999999999,27.4362251590507,30.0096109045284));
#12037=CARTESIAN_POINT('',(-0.499999999999999,27.4362251590507,-5.56473183187052));
#12038=CARTESIAN_POINT('',(2.5,27.4362251590507,30.0096109045284));
#12039=CARTESIAN_POINT('',(-6.5,27.4362251590507,30.0096109045284));
#12040=CARTESIAN_POINT('',(2.5,27.4362251590507,26.0483789742253));
#12041=CARTESIAN_POINT('',(2.5,27.4362251590507,3.24030798257579));
#12042=CARTESIAN_POINT('',(1.,27.4362251590507,26.0483789742253));
#12043=CARTESIAN_POINT('Origin',(-16.5,18.4317729825679,48.8862095951938));
#12044=CARTESIAN_POINT('',(3.5,18.4317729825679,46.8862095951938));
#12045=CARTESIAN_POINT('',(-0.499999999999999,18.4317729825679,46.8862095951938));
#12046=CARTESIAN_POINT('',(-11.5,18.4317729825679,46.8862095951938));
#12047=CARTESIAN_POINT('',(3.5,18.4317729825679,48.8862095951938));
#12048=CARTESIAN_POINT('',(3.5,18.4317729825679,48.8862095951938));
#12049=CARTESIAN_POINT('',(-0.499999999999999,18.4317729825679,48.8862095951938));
#12050=CARTESIAN_POINT('',(-11.5,18.4317729825679,48.8862095951938));
#12051=CARTESIAN_POINT('',(-0.499999999999999,18.4317729825679,30.402562452839));
#12052=CARTESIAN_POINT('Origin',(5.5,16.4317729825678,48.8862095951938));
#12053=CARTESIAN_POINT('',(5.5,-3.56822701743215,46.8862095951938));
#12054=CARTESIAN_POINT('',(5.5,16.4317729825678,46.8862095951938));
#12055=CARTESIAN_POINT('',(5.5,18.8635459651357,46.8862095951938));
#12056=CARTESIAN_POINT('',(5.5,-3.56822701743215,48.8862095951938));
#12057=CARTESIAN_POINT('',(5.5,-3.56822701743215,48.8862095951938));
#12058=CARTESIAN_POINT('',(5.5,16.4317729825678,48.8862095951938));
#12059=CARTESIAN_POINT('',(5.5,18.8635459651357,48.8862095951938));
#12060=CARTESIAN_POINT('',(5.5,16.4317729825678,48.8862095951938));
#12061=CARTESIAN_POINT('Origin',(3.5,16.4317729825679,48.8862095951938));
#12062=CARTESIAN_POINT('Origin',(3.5,16.4317729825679,46.8862095951938));
#12063=CARTESIAN_POINT('Origin',(3.5,16.4317729825679,48.8862095951938));
#12064=CARTESIAN_POINT('Origin',(3.5,-5.56822701743215,48.8862095951938));
#12065=CARTESIAN_POINT('',(3.5,-5.56822701743215,46.8862095951938));
#12066=CARTESIAN_POINT('',(-1.5,-5.56822701743215,46.8862095951938));
#12067=CARTESIAN_POINT('',(3.5,-5.56822701743215,48.8862095951938));
#12068=CARTESIAN_POINT('',(-1.5,-5.56822701743215,48.8862095951938));
#12069=CARTESIAN_POINT('',(3.5,-5.56822701743215,48.8862095951938));
#12070=CARTESIAN_POINT('Origin',(3.5,-3.56822701743215,48.8862095951938));
#12071=CARTESIAN_POINT('Origin',(3.5,-3.56822701743215,46.8862095951938));
#12072=CARTESIAN_POINT('Origin',(3.5,-3.56822701743215,48.8862095951938));
#12073=CARTESIAN_POINT('Origin',(-6.5,21.2953189477036,48.8862095951938));
#12074=CARTESIAN_POINT('',(7.5,-6.43177298256785,48.8862095951938));
#12075=CARTESIAN_POINT('',(-6.5,-6.43177298256785,48.8862095951938));
#12076=CARTESIAN_POINT('',(7.5,19.2953189477036,48.8862095951938));
#12077=CARTESIAN_POINT('',(7.5,15.3987725179725,48.8862095951938));
#12078=CARTESIAN_POINT('',(-0.499999999999999,19.2953189477036,48.8862095951938));
#12079=CARTESIAN_POINT('',(-6.5,19.2953189477036,48.8862095951938));
#12080=CARTESIAN_POINT('',(-0.499999999999999,2.03522655283679,48.8862095951938));
#12081=CARTESIAN_POINT('Origin',(-0.499999999999999,9.50222608824143,11.9189153104842));
#12082=CARTESIAN_POINT('',(-0.499999999999999,25.4362251590507,-20.9723835636495));
#12083=CARTESIAN_POINT('Origin',(-0.499999999999999,25.0098518119976,-22.4105093470644));
#12084=CARTESIAN_POINT('',(-0.499999999999999,25.4362251590507,28.1301265480575));
#12085=CARTESIAN_POINT('',(-0.499999999999999,25.4362251590507,-5.56473183187052));
#12086=CARTESIAN_POINT('',(-0.499999999999999,23.5204710981556,30.0096109045284));
#12087=CARTESIAN_POINT('Origin',(-0.499999999999999,24.9477990585308,29.5483789742253));
#12088=CARTESIAN_POINT('',(-0.499999999999999,22.2953189477036,30.0096109045284));
#12089=CARTESIAN_POINT('',(-0.499999999999999,17.4692256236461,30.0096109045284));
#12090=CARTESIAN_POINT('',(-0.499999999999999,19.2953189477036,33.0096109045284));
#12091=CARTESIAN_POINT('Origin',(-0.499999999999999,22.2953189477035,33.0096109045284));
#12092=CARTESIAN_POINT('',(-0.499999999999999,19.2953189477036,46.8862095951938));
#12093=CARTESIAN_POINT('',(-0.499999999999999,19.2953189477035,22.4642631075063));
#12094=CARTESIAN_POINT('',(-0.499999999999999,15.3987725179725,46.8862095951938));
#12095=CARTESIAN_POINT('',(-0.499999999999999,21.2953189477036,46.8862095951938));
#12096=CARTESIAN_POINT('Origin',(-0.499999999999999,19.2953189477036,46.8862095951938));
#12097=CARTESIAN_POINT('',(-0.499999999999999,21.2953189477036,33.0096109045284));
#12098=CARTESIAN_POINT('',(-0.499999999999999,21.2953189477035,22.4642631075063));
#12099=CARTESIAN_POINT('',(-0.499999999999999,22.2953189477036,32.0096109045284));
#12100=CARTESIAN_POINT('Origin',(-0.499999999999999,22.2953189477035,33.0096109045284));
#12101=CARTESIAN_POINT('',(-0.499999999999999,25.4362251590507,32.0096109045284));
#12102=CARTESIAN_POINT('',(-0.499999999999999,17.4692256236461,32.0096109045284));
#12103=CARTESIAN_POINT('Origin',(-0.499999999999999,25.4362251590507,30.0096109045284));
#12104=CARTESIAN_POINT('',(-0.499999999999999,25.4362251590507,-25.0483789742253));
#12105=CARTESIAN_POINT('Origin',(-0.499999999999999,25.4362251590507,-23.0483789742253));
#12106=CARTESIAN_POINT('',(-0.499999999999999,1.53522655283679,-25.0483789742253));
#12107=CARTESIAN_POINT('Origin',(8.5,24.9477990585308,29.5483789742253));
#12108=CARTESIAN_POINT('',(2.5,23.4477990585308,29.5483789742253));
#12109=CARTESIAN_POINT('Origin',(2.5,24.9477990585308,29.5483789742253));
#12110=CARTESIAN_POINT('',(0.499999999999999,23.4477990585308,29.5483789742253));
#12111=CARTESIAN_POINT('',(8.5,23.4477990585308,29.5483789742253));
#12112=CARTESIAN_POINT('',(0.499999999999999,23.5204710981556,30.0096109045284));
#12113=CARTESIAN_POINT('Origin',(0.499999999999999,24.9477990585308,29.5483789742253));
#12114=CARTESIAN_POINT('',(8.5,23.5204710981556,30.0096109045284));
#12115=CARTESIAN_POINT('',(0.499999999999999,25.4362251590507,28.1301265480575));
#12116=CARTESIAN_POINT('',(8.5,25.4362251590507,28.1301265480575));
#12117=CARTESIAN_POINT('Origin',(0.499999999999999,24.9477990585308,29.5483789742253));
#12118=CARTESIAN_POINT('Origin',(8.5,25.0098518119976,-22.4105093470644));
#12119=CARTESIAN_POINT('',(2.5,23.5098518119976,-22.4105093470644));
#12120=CARTESIAN_POINT('Origin',(2.5,25.0098518119976,-22.4105093470644));
#12121=CARTESIAN_POINT('',(0.499999999999999,23.5098518119976,-22.4105093470644));
#12122=CARTESIAN_POINT('',(8.5,23.5098518119976,-22.4105093470644));
#12123=CARTESIAN_POINT('',(0.499999999999999,25.4362251590507,-20.9723835636495));
#12124=CARTESIAN_POINT('Origin',(0.499999999999999,25.0098518119976,-22.4105093470644));
#12125=CARTESIAN_POINT('',(8.5,25.4362251590507,-20.9723835636495));
#12126=CARTESIAN_POINT('Origin',(0.499999999999999,25.0098518119976,-22.4105093470644));
#12127=CARTESIAN_POINT('Origin',(8.5,-5.94334688204796,29.5483789742253));
#12128=CARTESIAN_POINT('',(2.5,-7.44334688204796,29.5483789742253));
#12129=CARTESIAN_POINT('Origin',(2.5,-5.94334688204796,29.5483789742253));
#12130=CARTESIAN_POINT('',(8.5,-7.44334688204796,29.5483789742253));
#12131=CARTESIAN_POINT('',(0.499999999999999,-6.43177298256785,30.9666314003931));
#12132=CARTESIAN_POINT('',(8.5,-6.43177298256785,30.9666314003931));
#12133=CARTESIAN_POINT('',(0.499999999999999,-6.43177298256785,28.1301265480575));
#12134=CARTESIAN_POINT('Origin',(0.499999999999999,-5.94334688204796,29.5483789742253));
#12135=CARTESIAN_POINT('',(8.5,-6.43177298256785,28.1301265480575));
#12136=CARTESIAN_POINT('Origin',(8.5,-6.00539963551477,-22.4105093470644));
#12137=CARTESIAN_POINT('',(2.5,-7.50539963551477,-22.4105093470644));
#12138=CARTESIAN_POINT('Origin',(2.5,-6.00539963551477,-22.4105093470644));
#12139=CARTESIAN_POINT('',(8.5,-7.50539963551477,-22.4105093470644));
#12140=CARTESIAN_POINT('',(0.499999999999999,-6.43177298256785,-20.9723835636495));
#12141=CARTESIAN_POINT('',(8.5,-6.43177298256785,-20.9723835636495));
#12142=CARTESIAN_POINT('Origin',(0.499999999999999,-6.00539963551477,-22.4105093470644));
#12143=CARTESIAN_POINT('Origin',(-6.5,25.4362251590507,30.0096109045284));
#12144=CARTESIAN_POINT('',(0.499999999999999,22.2953189477036,30.0096109045284));
#12145=CARTESIAN_POINT('',(0.499999999999999,25.1891186339208,30.0096109045284));
#12146=CARTESIAN_POINT('',(-6.5,22.2953189477036,30.0096109045284));
#12147=CARTESIAN_POINT('Origin',(0.499999999999999,24.9730384855242,-22.4794441606449));
#12148=CARTESIAN_POINT('',(0.499999999999998,25.4362251590507,-17.9105093470644));
#12149=CARTESIAN_POINT('',(0.499999999999999,24.9914451487609,-17.9105093470644));
#12150=CARTESIAN_POINT('',(0.499999999999999,25.4362251590507,3.24030798257579));
#12151=CARTESIAN_POINT('Origin',(0.499999999999999,24.9420121087908,29.5289949393769));
#12152=CARTESIAN_POINT('',(0.499999999999999,-6.43177298256785,34.0483789742253));
#12153=CARTESIAN_POINT('',(0.499999999999999,-6.43177298256785,39.2172942847095));
#12154=CARTESIAN_POINT('',(0.499999999999999,-5.94334688204796,34.0483789742253));
#12155=CARTESIAN_POINT('',(0.499999999999999,-7.18466645743788,34.0483789742253));
#12156=CARTESIAN_POINT('',(0.499999999999999,-5.94334688204796,25.0483789742253));
#12157=CARTESIAN_POINT('Origin',(0.499999999999999,-5.94334688204796,29.5483789742253));
#12158=CARTESIAN_POINT('',(0.499999999999999,-6.43177298256785,25.0483789742253));
#12159=CARTESIAN_POINT('',(0.499999999999999,-5.94045340717793,25.0483789742253));
#12160=CARTESIAN_POINT('',(0.499999999999999,-6.43177298256785,39.2172942847095));
#12161=CARTESIAN_POINT('Origin',(-6.5,-6.43177298256785,48.8862095951938));
#12162=CARTESIAN_POINT('',(6.5,-6.43177298256785,46.8862095951938));
#12163=CARTESIAN_POINT('',(-6.5,-6.43177298256785,46.8862095951938));
#12164=CARTESIAN_POINT('',(6.5,-6.43177298256785,34.0483789742253));
#12165=CARTESIAN_POINT('',(6.5,-6.43177298256785,30.402562452839));
#12166=CARTESIAN_POINT('',(1.,-6.43177298256785,34.0483789742253));
#12167=CARTESIAN_POINT('Origin',(-6.5,-6.43177298256785,48.8862095951938));
#12168=CARTESIAN_POINT('',(6.5,-6.43177298256785,25.0483789742253));
#12169=CARTESIAN_POINT('',(1.,-6.43177298256785,25.0483789742253));
#12170=CARTESIAN_POINT('',(6.5,-6.43177298256785,-17.9105093470644));
#12171=CARTESIAN_POINT('',(6.5,-6.43177298256785,30.402562452839));
#12172=CARTESIAN_POINT('',(0.499999999999998,-6.43177298256785,-17.9105093470644));
#12173=CARTESIAN_POINT('',(1.,-6.43177298256785,-17.9105093470644));
#12174=CARTESIAN_POINT('',(0.499999999999999,-6.43177298256785,13.2033827172745));
#12175=CARTESIAN_POINT('Origin',(8.5,-8.43177298256785,34.0483789742253));
#12176=CARTESIAN_POINT('',(6.5,-5.94334688204796,34.0483789742253));
#12177=CARTESIAN_POINT('',(6.5,0.535226552836791,34.0483789742253));
#12178=CARTESIAN_POINT('',(8.5,-5.94334688204796,34.0483789742253));
#12179=CARTESIAN_POINT('Origin',(-6.5,21.2953189477036,46.8862095951938));
#12180=CARTESIAN_POINT('',(6.5,19.2953189477036,46.8862095951938));
#12181=CARTESIAN_POINT('',(-6.5,19.2953189477036,46.8862095951938));
#12182=CARTESIAN_POINT('',(6.5,15.3987725179725,46.8862095951938));
#12183=CARTESIAN_POINT('Origin',(6.5,9.50222608824143,11.9189153104842));
#12184=CARTESIAN_POINT('',(6.5,20.5630459545133,30.5602782858212));
#12185=CARTESIAN_POINT('',(6.5,24.9477990585308,25.0483789742253));
#12186=CARTESIAN_POINT('Origin',(6.5,24.9477990585308,29.5483789742253));
#12187=CARTESIAN_POINT('',(6.5,25.4362251590507,25.0483789742253));
#12188=CARTESIAN_POINT('',(6.5,18.4692256236461,25.0483789742253));
#12189=CARTESIAN_POINT('',(6.5,25.4362251590507,-17.9105093470644));
#12190=CARTESIAN_POINT('',(6.5,25.4362251590507,-5.56473183187052));
#12191=CARTESIAN_POINT('',(6.5,17.2560389501195,-17.9105093470644));
#12192=CARTESIAN_POINT('',(6.5,-1.50539963551477,-22.4105093470644));
#12193=CARTESIAN_POINT('',(6.5,-1.50539963551477,-5.2457970182901));
#12194=CARTESIAN_POINT('',(6.5,-6.00539963551477,-17.9105093470644));
#12195=CARTESIAN_POINT('Origin',(6.5,-6.00539963551477,-22.4105093470644));
#12196=CARTESIAN_POINT('',(6.5,0.535226552836792,-17.9105093470644));
#12197=CARTESIAN_POINT('',(6.5,-5.94334688204796,25.0483789742253));
#12198=CARTESIAN_POINT('',(6.5,18.4692256236461,25.0483789742253));
#12199=CARTESIAN_POINT('Origin',(6.5,-5.94334688204796,29.5483789742253));
#12200=CARTESIAN_POINT('',(6.5,19.2953189477036,33.0096109045284));
#12201=CARTESIAN_POINT('',(6.5,19.2953189477035,22.4642631075063));
#12202=CARTESIAN_POINT('Origin',(6.5,22.2953189477035,33.0096109045284));
#12203=CARTESIAN_POINT('Origin',(-6.5,19.2953189477036,33.0096109045284));
#12204=CARTESIAN_POINT('',(-6.5,19.2953189477036,33.0096109045284));
#12205=CARTESIAN_POINT('Origin',(-6.5,22.2953189477035,33.0096109045284));
#12206=CARTESIAN_POINT('',(0.499999999999999,20.5630459545133,30.5602782858212));
#12207=CARTESIAN_POINT('Origin',(0.499999999999999,22.2953189477035,33.0096109045284));
#12208=CARTESIAN_POINT('',(8.5,20.5630459545133,30.5602782858212));
#12209=CARTESIAN_POINT('Origin',(8.5,24.9477990585308,29.5483789742253));
#12210=CARTESIAN_POINT('',(0.499999999999999,24.9477990585308,25.0483789742253));
#12211=CARTESIAN_POINT('Origin',(0.499999999999999,24.9477990585308,29.5483789742253));
#12212=CARTESIAN_POINT('',(8.5,24.9477990585308,25.0483789742253));
#12213=CARTESIAN_POINT('Origin',(8.5,27.4362251590507,25.0483789742253));
#12214=CARTESIAN_POINT('',(8.5,-5.94334688204796,25.0483789742253));
#12215=CARTESIAN_POINT('Origin',(8.5,27.4362251590507,25.0483789742253));
#12216=CARTESIAN_POINT('',(0.499999999999999,25.4362251590507,25.0483789742253));
#12217=CARTESIAN_POINT('',(0.499999999999999,26.1891186339208,25.0483789742253));
#12218=CARTESIAN_POINT('',(1.,25.4362251590507,25.0483789742253));
#12219=CARTESIAN_POINT('Origin',(0.499999999999999,24.9420121087908,29.5289949393769));
#12220=CARTESIAN_POINT('',(0.499999999999999,25.4362251590507,3.24030798257579));
#12221=CARTESIAN_POINT('Origin',(-6.5,25.4362251590507,-23.0483789742253));
#12222=CARTESIAN_POINT('',(1.,25.4362251590507,-17.9105093470644));
#12223=CARTESIAN_POINT('Origin',(8.5,-5.94334688204796,29.5483789742253));
#12224=CARTESIAN_POINT('Origin',(8.5,25.0098518119976,-17.9105093470644));
#12225=CARTESIAN_POINT('',(0.499999999999999,-6.00539963551477,-17.9105093470644));
#12226=CARTESIAN_POINT('',(8.5,-6.00539963551477,-17.9105093470644));
#12227=CARTESIAN_POINT('',(0.499999999999999,-7.20017964580458,-17.9105093470644));
#12228=CARTESIAN_POINT('Origin',(8.5,-1.50539963551477,-22.4105093470644));
#12229=CARTESIAN_POINT('',(0.499999999999999,-1.50539963551477,-22.4105093470644));
#12230=CARTESIAN_POINT('',(0.499999999999999,-1.50539963551477,-22.4449767538547));
#12231=CARTESIAN_POINT('',(8.5,-1.50539963551477,-22.4105093470644));
#12232=CARTESIAN_POINT('Origin',(8.5,-6.00539963551477,-22.4105093470644));
#12233=CARTESIAN_POINT('Origin',(0.499999999999999,-6.00539963551477,-22.4105093470644));
#12234=CARTESIAN_POINT('Origin',(0.499999999999999,-5.96858630904131,-22.4794441606449));
#12235=CARTESIAN_POINT('Origin',(8.5,25.0098518119976,-17.9105093470644));
#12236=CARTESIAN_POINT('Origin',(7.5,0.535226552836791,33.0483789742253));
#12237=CARTESIAN_POINT('',(7.5,-7.43177298256785,32.0483789742253));
#12238=CARTESIAN_POINT('Origin',(7.5,-7.43177298256785,33.0483789742253));
#12239=CARTESIAN_POINT('',(7.5,-5.94334688204796,32.0483789742253));
#12240=CARTESIAN_POINT('',(7.5,0.535226552836791,32.0483789742253));
#12241=CARTESIAN_POINT('Origin',(7.5,-5.94334688204796,33.0483789742253));
#12242=CARTESIAN_POINT('Origin',(7.5,-5.94334688204796,29.5483789742253));
#12243=CARTESIAN_POINT('',(7.5,-5.94334688204796,27.0483789742253));
#12244=CARTESIAN_POINT('Origin',(7.5,-5.94334688204796,26.0483789742253));
#12245=CARTESIAN_POINT('Origin',(7.5,-5.94334688204796,29.5483789742253));
#12246=CARTESIAN_POINT('Origin',(7.5,1.77943960309674,26.0483789742253));
#12247=CARTESIAN_POINT('',(7.5,-7.43177298256785,27.0483789742253));
#12248=CARTESIAN_POINT('Origin',(7.5,-7.43177298256785,26.0483789742253));
#12249=CARTESIAN_POINT('',(7.5,1.77943960309674,27.0483789742253));
#12250=CARTESIAN_POINT('Origin',(7.5,22.2953189477035,33.0096109045284));
#12251=CARTESIAN_POINT('',(7.5,22.046233320739,32.041129438294));
#12252=CARTESIAN_POINT('Origin',(7.5,21.7971476937744,31.0726479720595));
#12253=CARTESIAN_POINT('',(7.5,21.2953189477036,33.0096109045284));
#12254=CARTESIAN_POINT('Origin',(7.5,22.2953189477035,33.0096109045284));
#12255=CARTESIAN_POINT('Origin',(7.5,20.2953189477035,33.0096109045284));
#12256=CARTESIAN_POINT('Origin',(7.5,20.2953189477035,22.4642631075063));
#12257=CARTESIAN_POINT('',(7.5,21.2953189477036,46.8862095951938));
#12258=CARTESIAN_POINT('Origin',(7.5,20.2953189477035,46.8862095951938));
#12259=CARTESIAN_POINT('',(7.5,21.2953189477035,22.4642631075063));
#12260=CARTESIAN_POINT('Ctrl Pts',(8.5,19.2953189477036,47.8862095951938));
#12261=CARTESIAN_POINT('Ctrl Pts',(8.5,20.2953189477035,47.8862095951938));
#12262=CARTESIAN_POINT('Ctrl Pts',(8.5,20.2953189477035,46.8862095951938));
#12263=CARTESIAN_POINT('Ctrl Pts',(8.5,19.2953189477036,48.8862095951938));
#12264=CARTESIAN_POINT('Ctrl Pts',(8.5,21.2953189477035,48.8862095951938));
#12265=CARTESIAN_POINT('Ctrl Pts',(8.5,21.2953189477035,46.8862095951938));
#12266=CARTESIAN_POINT('Ctrl Pts',(7.5,19.2953189477036,48.8862095951938));
#12267=CARTESIAN_POINT('Ctrl Pts',(7.5,21.2953189477035,48.8862095951938));
#12268=CARTESIAN_POINT('Ctrl Pts',(7.5,21.2953189477035,46.8862095951938));
#12269=CARTESIAN_POINT('Origin',(7.5,19.2953189477036,47.8862095951938));
#12270=CARTESIAN_POINT('Origin',(7.5,19.2953189477036,46.8862095951938));
#12271=CARTESIAN_POINT('Origin',(7.5,15.3987725179725,47.8862095951938));
#12272=CARTESIAN_POINT('Origin',(7.5,-6.43177298256785,47.8862095951938));
#12273=CARTESIAN_POINT('Ctrl Pts',(8.5,-7.43177298256785,46.8862095951938));
#12274=CARTESIAN_POINT('Ctrl Pts',(8.5,-7.43177298256785,47.8862095951938));
#12275=CARTESIAN_POINT('Ctrl Pts',(8.5,-6.43177298256785,47.8862095951938));
#12276=CARTESIAN_POINT('Ctrl Pts',(8.5,-8.43177298256784,46.8862095951938));
#12277=CARTESIAN_POINT('Ctrl Pts',(8.5,-8.43177298256784,48.8862095951938));
#12278=CARTESIAN_POINT('Ctrl Pts',(8.5,-6.43177298256785,48.8862095951938));
#12279=CARTESIAN_POINT('Ctrl Pts',(7.5,-8.43177298256784,46.8862095951938));
#12280=CARTESIAN_POINT('Ctrl Pts',(7.5,-8.43177298256784,48.8862095951938));
#12281=CARTESIAN_POINT('Ctrl Pts',(7.5,-6.43177298256785,48.8862095951938));
#12282=CARTESIAN_POINT('Origin',(7.5,-7.43177298256785,46.8862095951938));
#12283=CARTESIAN_POINT('Origin',(7.5,-6.43177298256785,46.8862095951938));
#12284=CARTESIAN_POINT('Origin',(7.5,-7.43177298256785,30.402562452839));
#12285=CARTESIAN_POINT('Origin',(7.5,-7.43177298256785,33.0483789742253));
#12286=CARTESIAN_POINT('Origin',(7.5,18.4692256236461,26.0483789742253));
#12287=CARTESIAN_POINT('',(7.5,26.4362251590507,27.0483789742253));
#12288=CARTESIAN_POINT('Origin',(7.5,26.4362251590507,26.0483789742253));
#12289=CARTESIAN_POINT('',(7.5,24.9477990585308,27.0483789742253));
#12290=CARTESIAN_POINT('',(7.5,18.4692256236461,27.0483789742253));
#12291=CARTESIAN_POINT('Origin',(7.5,24.9477990585308,26.0483789742253));
#12292=CARTESIAN_POINT('Origin',(7.5,24.9477990585308,29.5483789742253));
#12293=CARTESIAN_POINT('',(7.5,22.6973337979905,30.6371425441069));
#12294=CARTESIAN_POINT('Origin',(7.5,21.7971476937744,31.0726479720595));
#12295=CARTESIAN_POINT('Origin',(7.5,24.9477990585308,29.5483789742253));
#12296=CARTESIAN_POINT('Origin',(7.5,26.4362251590507,26.0483789742253));
#12297=CARTESIAN_POINT('Origin',(7.5,26.4362251590507,26.0483789742253));
#12298=CARTESIAN_POINT('Origin',(7.5,21.7971476937744,31.0726479720595));
#12299=CARTESIAN_POINT('Origin',(7.5,21.7971476937744,31.0726479720595));
#12300=CARTESIAN_POINT('Origin',(7.5,-7.43177298256785,33.0483789742253));
#12301=CARTESIAN_POINT('Origin',(7.5,-7.43177298256785,33.0483789742253));
#12302=CARTESIAN_POINT('Origin',(7.5,-7.43177298256785,26.0483789742253));
#12303=CARTESIAN_POINT('Origin',(7.5,-7.43177298256785,26.0483789742253));
#12304=CARTESIAN_POINT('Origin',(1.,-7.43177298256785,26.0483789742253));
#12305=CARTESIAN_POINT('',(2.5,-7.43177298256785,27.0483789742253));
#12306=CARTESIAN_POINT('',(1.,-7.43177298256785,27.0483789742253));
#12307=CARTESIAN_POINT('Origin',(2.5,-7.43177298256785,26.0483789742253));
#12308=CARTESIAN_POINT('Origin',(8.5,-5.94334688204796,27.0483789742253));
#12309=CARTESIAN_POINT('',(2.5,-5.94334688204796,27.0483789742253));
#12310=CARTESIAN_POINT('',(8.5,-5.94334688204796,27.0483789742253));
#12311=CARTESIAN_POINT('',(2.5,-5.94334688204796,27.0483789742253));
#12312=CARTESIAN_POINT('Origin',(8.5,-5.94334688204796,29.5483789742253));
#12313=CARTESIAN_POINT('',(2.5,-5.94334688204796,32.0483789742253));
#12314=CARTESIAN_POINT('',(8.5,-5.94334688204796,32.0483789742253));
#12315=CARTESIAN_POINT('Origin',(2.5,-5.94334688204796,29.5483789742253));
#12316=CARTESIAN_POINT('Origin',(8.5,-8.43177298256785,32.0483789742253));
#12317=CARTESIAN_POINT('',(2.5,-7.43177298256785,32.0483789742253));
#12318=CARTESIAN_POINT('',(1.,-7.43177298256785,32.0483789742253));
#12319=CARTESIAN_POINT('',(2.5,-5.94334688204796,32.0483789742253));
#12320=CARTESIAN_POINT('Origin',(1.,-7.43177298256785,33.0483789742253));
#12321=CARTESIAN_POINT('Origin',(2.5,-7.43177298256785,33.0483789742253));
#12322=CARTESIAN_POINT('Origin',(-6.5,-6.43177298256785,46.8862095951938));
#12323=CARTESIAN_POINT('Origin',(-6.5,19.2953189477036,46.8862095951938));
#12324=CARTESIAN_POINT('',(-6.5,21.2953189477036,46.8862095951938));
#12325=CARTESIAN_POINT('Origin',(-6.5,21.2953189477036,33.0096109045284));
#12326=CARTESIAN_POINT('',(-6.5,21.2953189477036,33.0096109045284));
#12327=CARTESIAN_POINT('Origin',(-6.5,22.2953189477035,33.0096109045284));
#12328=CARTESIAN_POINT('',(2.5,22.046233320739,32.041129438294));
#12329=CARTESIAN_POINT('',(-6.5,22.046233320739,32.041129438294));
#12330=CARTESIAN_POINT('',(2.5,22.2953189477036,32.0096109045284));
#12331=CARTESIAN_POINT('Origin',(2.5,22.2953189477035,33.0096109045284));
#12332=CARTESIAN_POINT('',(-6.5,22.2953189477036,32.0096109045284));
#12333=CARTESIAN_POINT('Origin',(-6.5,21.7971476937744,31.0726479720595));
#12334=CARTESIAN_POINT('',(2.5,22.6973337979905,30.6371425441069));
#12335=CARTESIAN_POINT('',(-6.5,22.6973337979905,30.6371425441069));
#12336=CARTESIAN_POINT('Origin',(2.5,21.7971476937744,31.0726479720595));
#12337=CARTESIAN_POINT('Origin',(8.5,24.9477990585308,29.5483789742253));
#12338=CARTESIAN_POINT('',(2.5,24.9477990585308,27.0483789742253));
#12339=CARTESIAN_POINT('',(8.5,24.9477990585308,27.0483789742253));
#12340=CARTESIAN_POINT('Origin',(2.5,24.9477990585308,29.5483789742253));
#12341=CARTESIAN_POINT('Origin',(8.5,27.4362251590507,27.0483789742253));
#12342=CARTESIAN_POINT('',(2.5,26.4362251590507,27.0483789742253));
#12343=CARTESIAN_POINT('',(1.,26.4362251590507,27.0483789742253));
#12344=CARTESIAN_POINT('',(2.5,24.9477990585308,27.0483789742253));
#12345=CARTESIAN_POINT('Origin',(1.,26.4362251590507,26.0483789742253));
#12346=CARTESIAN_POINT('Origin',(2.5,26.4362251590507,26.0483789742253));
#12347=CARTESIAN_POINT('Origin',(8.5,-8.43177298256785,-19.9105093470644));
#12348=CARTESIAN_POINT('',(2.5,-6.00539963551477,-19.9105093470644));
#12349=CARTESIAN_POINT('',(2.5,-6.00539963551477,-19.9105093470644));
#12350=CARTESIAN_POINT('',(8.5,-6.00539963551477,-19.9105093470644));
#12351=CARTESIAN_POINT('Origin',(8.5,-3.50539963551477,-22.4105093470644));
#12352=CARTESIAN_POINT('',(2.5,-3.50539963551477,-22.4105093470644));
#12353=CARTESIAN_POINT('',(8.5,-3.50539963551477,-22.4105093470644));
#12354=CARTESIAN_POINT('',(2.5,-3.50539963551477,-25.0483789742253));
#12355=CARTESIAN_POINT('',(2.5,-3.50539963551477,-22.4105093470644));
#12356=CARTESIAN_POINT('',(1.,-3.50539963551477,-25.0483789742253));
#12357=CARTESIAN_POINT('Origin',(8.5,-6.00539963551477,-22.4105093470644));
#12358=CARTESIAN_POINT('Origin',(2.5,-6.00539963551477,-22.4105093470644));
#12359=CARTESIAN_POINT('Origin',(2.5,-5.96858630904131,-22.4794441606449));
#12360=CARTESIAN_POINT('',(2.5,-6.43177298256785,-25.0483789742253));
#12361=CARTESIAN_POINT('Origin',(2.5,-6.43177298256785,-23.0483789742253));
#12362=CARTESIAN_POINT('',(2.5,-6.20017964580458,-25.0483789742253));
#12363=CARTESIAN_POINT('Origin',(2.5,24.9420121087908,29.5289949393769));
#12364=CARTESIAN_POINT('',(2.5,25.4362251590507,32.0096109045284));
#12365=CARTESIAN_POINT('',(2.5,25.1891186339208,32.0096109045284));
#12366=CARTESIAN_POINT('Origin',(2.5,25.4362251590507,30.0096109045284));
#12367=CARTESIAN_POINT('Origin',(8.5,25.0098518119976,-19.9105093470644));
#12368=CARTESIAN_POINT('',(2.5,25.0098518119976,-19.9105093470644));
#12369=CARTESIAN_POINT('',(8.5,25.0098518119976,-19.9105093470644));
#12370=CARTESIAN_POINT('',(2.5,25.0098518119976,-19.9105093470644));
#12371=CARTESIAN_POINT('Origin',(8.5,25.0098518119976,-22.4105093470644));
#12372=CARTESIAN_POINT('',(2.5,22.5098518119976,-22.4105093470644));
#12373=CARTESIAN_POINT('',(8.5,22.5098518119976,-22.4105093470644));
#12374=CARTESIAN_POINT('Origin',(2.5,25.0098518119976,-22.4105093470644));
#12375=CARTESIAN_POINT('Origin',(8.5,22.5098518119976,-25.0483789742253));
#12376=CARTESIAN_POINT('',(2.5,22.5098518119976,-25.0483789742253));
#12377=CARTESIAN_POINT('',(1.,22.5098518119976,-25.0483789742253));
#12378=CARTESIAN_POINT('',(2.5,22.5098518119976,-22.4105093470644));
#12379=CARTESIAN_POINT('Origin',(2.5,24.9730384855242,-22.4794441606449));
#12380=CARTESIAN_POINT('',(2.5,25.4362251590507,-25.0483789742253));
#12381=CARTESIAN_POINT('',(2.5,9.27063275147817,-25.0483789742253));
#12382=CARTESIAN_POINT('Origin',(2.5,25.4362251590507,-23.0483789742253));
#12383=CARTESIAN_POINT('Origin',(2.5,-5.93755993230791,29.5483789742253));
#12384=CARTESIAN_POINT('Origin',(-6.5,25.4362251590507,32.0096109045284));
#12385=CARTESIAN_POINT('',(-6.5,25.4362251590507,32.0096109045284));
#12386=CARTESIAN_POINT('Origin',(-6.5,-6.43177298256785,-25.0483789742253));
#12387=CARTESIAN_POINT('',(-6.5,25.4362251590507,-25.0483789742253));
#12388=CARTESIAN_POINT('',(-6.5,-6.43177298256785,-25.0483789742253));
#12389=CARTESIAN_POINT('Origin',(-6.5,25.4362251590507,30.0096109045284));
#12390=CARTESIAN_POINT('Origin',(-6.5,25.4362251590507,-23.0483789742253));
#12391=CARTESIAN_POINT('Origin',(-6.5,-6.43177298256785,-23.0483789742253));
#17016=UNCERTAINTY_MEASURE_WITH_UNIT(LENGTH_MEASURE(0.01),#17043,
'DISTANCE_ACCURACY_VALUE',
'Maximum model space distance between geometric entities at asserted c
onnectivities');
#17028=UNCERTAINTY_MEASURE_WITH_UNIT(LENGTH_MEASURE(0.01),#17043,
'DISTANCE_ACCURACY_VALUE',
'Maximum model space distance between geometric entities at asserted c
onnectivities');
#17030=(
GEOMETRIC_REPRESENTATION_CONTEXT(3)
GLOBAL_UNCERTAINTY_ASSIGNED_CONTEXT((#17016))
GLOBAL_UNIT_ASSIGNED_CONTEXT((#17043,#17045,#17046))
REPRESENTATION_CONTEXT('','3D')
);
#17042=(
GEOMETRIC_REPRESENTATION_CONTEXT(3)
GLOBAL_UNCERTAINTY_ASSIGNED_CONTEXT((#17028))
GLOBAL_UNIT_ASSIGNED_CONTEXT((#17043,#17045,#17046))
REPRESENTATION_CONTEXT('','3D')
);
#17043=(
LENGTH_UNIT()
NAMED_UNIT(*)
SI_UNIT(.MILLI.,.METRE.)
);
#17045=(
NAMED_UNIT(*)
PLANE_ANGLE_UNIT()
SI_UNIT($,.RADIAN.)
);
#17046=(
NAMED_UNIT(*)
SI_UNIT($,.STERADIAN.)
SOLID_ANGLE_UNIT()
);
#17048=SHAPE_DEFINITION_REPRESENTATION(#17061,#17086);
#17061=PRODUCT_DEFINITION_SHAPE('',$,#17100);
#17086=SHAPE_REPRESENTATION('',(#8261),#17030);
#17098=PRODUCT_DEFINITION_CONTEXT('part definition',#17139,'design');
#17100=PRODUCT_DEFINITION('CLAMSHELL_TOP','CLAMSHELL_TOP',#17113,#17098);
#17113=PRODUCT_DEFINITION_FORMATION('',$,#17142);
#17139=APPLICATION_CONTEXT(
'Core Data for Automotive Mechanical Design Process');
#17140=PRODUCT_CONTEXT('part definition',#17139,'mechanical');
#17142=PRODUCT('CLAMSHELL_TOP','CLAMSHELL_TOP',$,(#17140));
#17154=PRESENTATION_STYLE_ASSIGNMENT((#17155));
#17155=SURFACE_STYLE_USAGE(.BOTH.,#17156);
#17156=SURFACE_SIDE_STYLE('',(#17157));
#17157=SURFACE_STYLE_FILL_AREA(#17158);
#17158=FILL_AREA_STYLE('Steel - Satin',(#17159));
#17159=FILL_AREA_STYLE_COLOUR('Steel - Satin',#17160);
#17160=COLOUR_RGB('Steel - Satin', 0.09019608, 0.27058824, 0.51372549);
ENDSEC;
END-ISO-10303-21;
